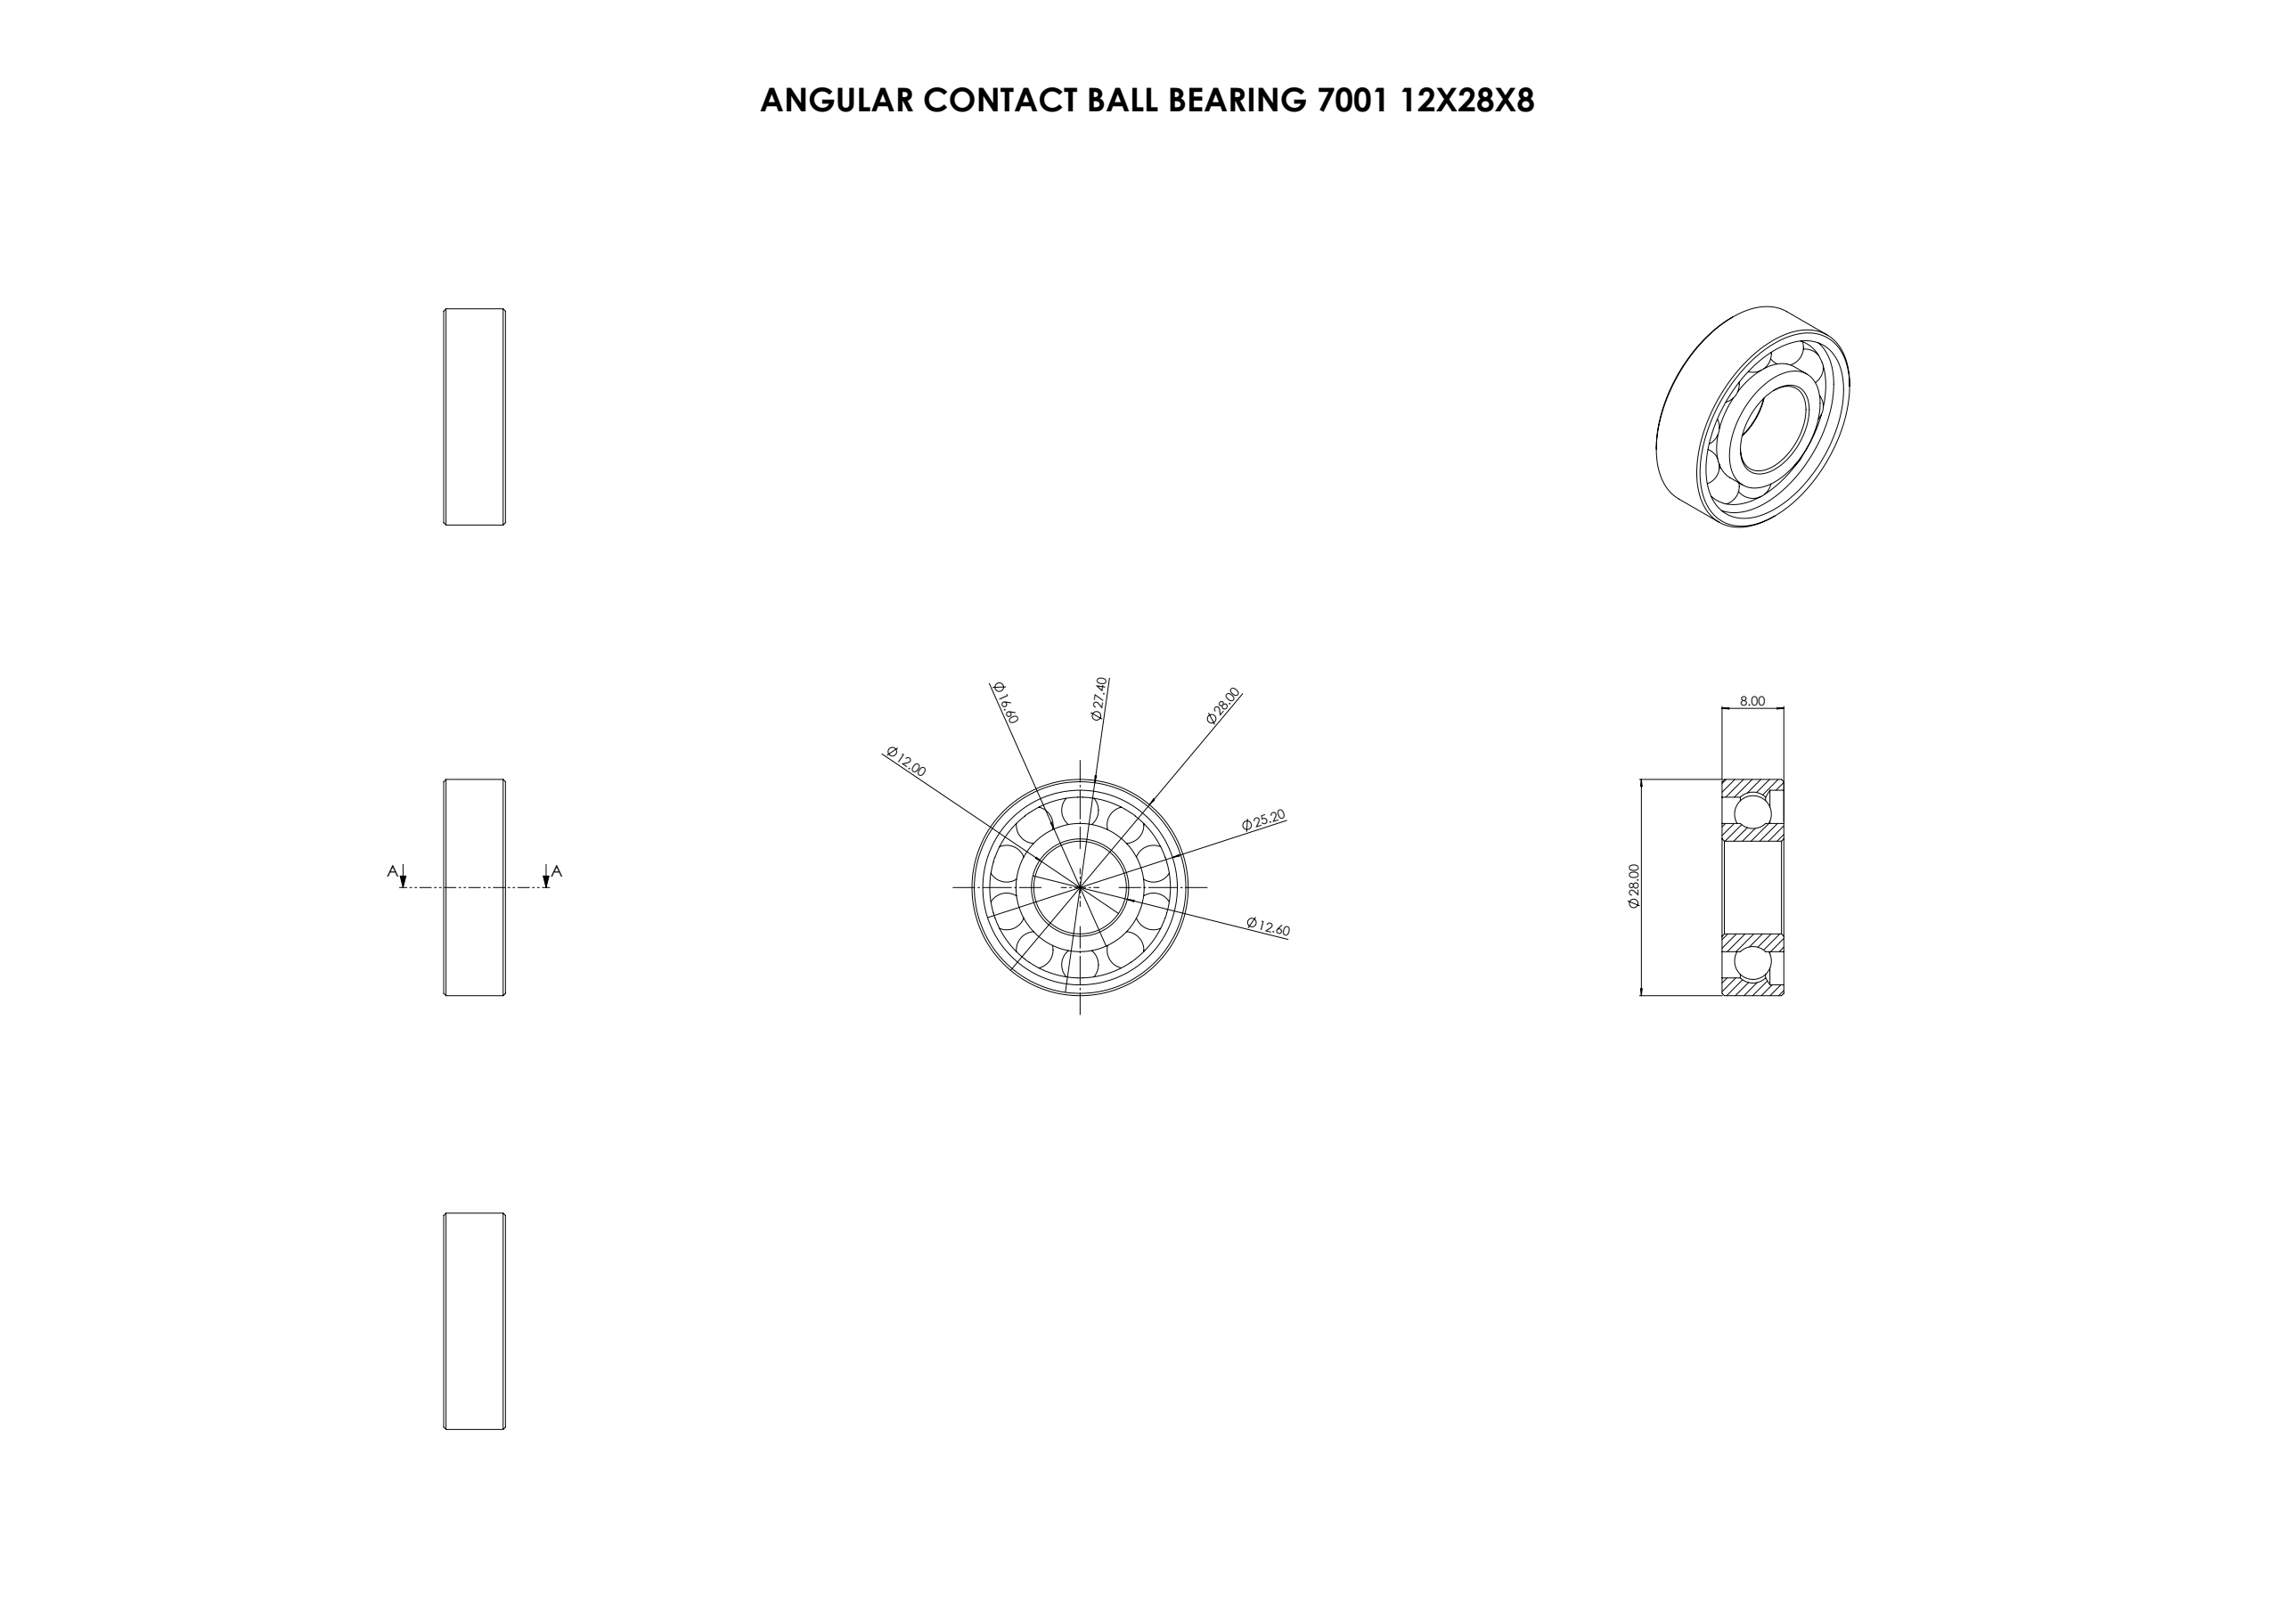
ISO-10303-21;
HEADER;
/* Generated by software containing ST-Developer
 * from STEP Tools, Inc. (www.steptools.com) 
 */

FILE_DESCRIPTION(
/* description */ (''),
/* implementation_level */ '2;1');

FILE_NAME(
/* name */ '06_Angular_Contact_Ball_Bearing_7001_12x28x8.step',
/* time_stamp */ '2026-10-11T09:12:28-07:00',
/* author */ (''),
/* organization */ (''),
/* preprocessor_version */ 'ST-DEVELOPER v20.2',
/* originating_system */ 'Autodesk Translation Framework v15.15.0.0',
/* authorisation */ '');

FILE_SCHEMA (('AUTOMOTIVE_DESIGN { 1 0 10303 214 3 1 1 }'));
ENDSEC;

DATA;
#10=MECHANICAL_DESIGN_GEOMETRIC_PRESENTATION_REPRESENTATION('',(#652),#23254);
#83=SPHERICAL_SURFACE('',#7605,2.38125);
#84=SPHERICAL_SURFACE('',#7635,2.38125);
#85=SPHERICAL_SURFACE('',#7641,2.38125);
#86=SPHERICAL_SURFACE('',#7647,2.38125);
#87=SPHERICAL_SURFACE('',#7653,2.38125);
#88=SPHERICAL_SURFACE('',#7659,2.38125);
#89=SPHERICAL_SURFACE('',#7665,2.38125);
#90=SPHERICAL_SURFACE('',#7671,2.38125);
#91=SPHERICAL_SURFACE('',#7677,2.38125);
#92=SPHERICAL_SURFACE('',#7689,2.38125);
#517=B_SPLINE_CURVE_WITH_KNOTS('',3,(#21115,#21116,#21117,#21118,#21119,
#21120),.UNSPECIFIED.,.F.,.F.,(4,2,4),(0.226218361876484,0.25919316472602,
0.292167967575556),.UNSPECIFIED.);
#518=B_SPLINE_CURVE_WITH_KNOTS('',3,(#21122,#21123,#21124,#21125,#21126,
#21127,#21128,#21129,#21130,#21131,#21132),.UNSPECIFIED.,.F.,.F.,(4,2,3,
2,4),(-0.170336741191592,-0.0873737681171707,0.,0.0873737681171706,0.170336741191592),
 .UNSPECIFIED.);
#519=B_SPLINE_CURVE_WITH_KNOTS('',3,(#21134,#21135,#21136,#21137,#21138,
#21139),.UNSPECIFIED.,.F.,.F.,(4,2,4),(0.958318332016868,0.991720601129839,
1.02512287024281),.UNSPECIFIED.);
#520=B_SPLINE_CURVE_WITH_KNOTS('',3,(#21140,#21141,#21142,#21143,#21144,
#21145,#21146,#21147,#21148,#21149,#21150),.UNSPECIFIED.,.F.,.F.,(4,2,3,
2,4),(-0.170336741191593,-0.0873737681171707,0.,0.0873737681171707,0.170336741191592),
 .UNSPECIFIED.);
#521=B_SPLINE_CURVE_WITH_KNOTS('',3,(#21153,#21154,#21155,#21156,#21157,
#21158),.UNSPECIFIED.,.F.,.F.,(4,2,4),(0.699168310489759,0.727019400778947,
0.754870491068134),.UNSPECIFIED.);
#522=B_SPLINE_CURVE_WITH_KNOTS('',3,(#21160,#21161,#21162,#21163,#21164,
#21165,#21166,#21167,#21168,#21169),.UNSPECIFIED.,.F.,.F.,(4,2,2,2,4),(0.528720639901106,
0.611686436801216,0.699059005116263,0.78643157343131,0.869397370331421),
 .UNSPECIFIED.);
#523=B_SPLINE_CURVE_WITH_KNOTS('',3,(#21171,#21172,#21173,#21174,#21175,
#21176),.UNSPECIFIED.,.F.,.F.,(4,2,4),(0.21448870997046,0.242339800259649,
0.270190890548838),.UNSPECIFIED.);
#524=B_SPLINE_CURVE_WITH_KNOTS('',3,(#21177,#21178,#21179,#21180,#21181,
#21182,#21183,#21184,#21185,#21186),.UNSPECIFIED.,.F.,.F.,(4,2,2,2,4),(0.528720639901106,
0.611686436801217,0.699059005116263,0.78643157343131,0.869397370331421),
 .UNSPECIFIED.);
#525=B_SPLINE_CURVE_WITH_KNOTS('',3,(#21193,#21194,#21195,#21196),
 .UNSPECIFIED.,.F.,.F.,(4,4),(0.991720601129836,1.02512287024281),
 .UNSPECIFIED.);
#526=B_SPLINE_CURVE_WITH_KNOTS('',3,(#21200,#21201,#21202,#21203,#21204,
#21205),.UNSPECIFIED.,.F.,.F.,(4,2,4),(0.958318332016865,0.991720601129836,
1.02512287024281),.UNSPECIFIED.);
#527=B_SPLINE_CURVE_WITH_KNOTS('',3,(#21209,#21210,#21211,#21212,#21213,
#21214),.UNSPECIFIED.,.F.,.F.,(4,2,4),(0.958318332016865,0.991720601129836,
1.02512287024281),.UNSPECIFIED.);
#528=B_SPLINE_CURVE_WITH_KNOTS('',3,(#21218,#21219,#21220,#21221,#21222,
#21223),.UNSPECIFIED.,.F.,.F.,(4,2,4),(0.958318332016865,0.991720601129836,
1.02512287024281),.UNSPECIFIED.);
#529=B_SPLINE_CURVE_WITH_KNOTS('',3,(#21227,#21228,#21229,#21230,#21231,
#21232),.UNSPECIFIED.,.F.,.F.,(4,2,4),(0.958318332016865,0.991720601129836,
1.02512287024281),.UNSPECIFIED.);
#530=B_SPLINE_CURVE_WITH_KNOTS('',3,(#21236,#21237,#21238,#21239,#21240,
#21241),.UNSPECIFIED.,.F.,.F.,(4,2,4),(0.958318332016865,0.991720601129836,
1.02512287024281),.UNSPECIFIED.);
#531=B_SPLINE_CURVE_WITH_KNOTS('',3,(#21246,#21247,#21248,#21249,#21250,
#21251),.UNSPECIFIED.,.F.,.F.,(4,2,4),(0.958318332016865,0.991720601129837,
1.02512287024281),.UNSPECIFIED.);
#532=B_SPLINE_CURVE_WITH_KNOTS('',3,(#21255,#21256,#21257,#21258,#21259,
#21260),.UNSPECIFIED.,.F.,.F.,(4,2,4),(0.958318332016865,0.991720601129836,
1.02512287024281),.UNSPECIFIED.);
#533=B_SPLINE_CURVE_WITH_KNOTS('',3,(#21264,#21265,#21266,#21267,#21268,
#21269),.UNSPECIFIED.,.F.,.F.,(4,2,4),(0.958318332016866,0.99172060112984,
1.02512287024281),.UNSPECIFIED.);
#534=B_SPLINE_CURVE_WITH_KNOTS('',3,(#21272,#21273,#21274,#21275),
 .UNSPECIFIED.,.F.,.F.,(4,4),(0.958318332016865,0.991720601129836),
 .UNSPECIFIED.);
#535=B_SPLINE_CURVE_WITH_KNOTS('',3,(#21279,#21280,#21281,#21282,#21283,
#21284,#21285,#21286,#21287,#21288,#21289),.UNSPECIFIED.,.F.,.F.,(4,2,3,
2,4),(-0.170336741191593,-0.0873737681171707,0.,0.0873737681171707,0.170336741191592),
 .UNSPECIFIED.);
#536=B_SPLINE_CURVE_WITH_KNOTS('',3,(#21294,#21295,#21296,#21297,#21298,
#21299),.UNSPECIFIED.,.F.,.F.,(4,2,4),(0.21448870997046,0.242339800259649,
0.270190890548838),.UNSPECIFIED.);
#537=B_SPLINE_CURVE_WITH_KNOTS('',3,(#21303,#21304,#21305,#21306,#21307,
#21308),.UNSPECIFIED.,.F.,.F.,(4,2,4),(0.21448870997046,0.242339800259649,
0.270190890548838),.UNSPECIFIED.);
#538=B_SPLINE_CURVE_WITH_KNOTS('',3,(#21312,#21313,#21314,#21315,#21316,
#21317),.UNSPECIFIED.,.F.,.F.,(4,2,4),(0.21448870997046,0.242339800259649,
0.270190890548838),.UNSPECIFIED.);
#539=B_SPLINE_CURVE_WITH_KNOTS('',3,(#21321,#21322,#21323,#21324),
 .UNSPECIFIED.,.F.,.F.,(4,4),(0.21448870997046,0.242339800259649),
 .UNSPECIFIED.);
#540=B_SPLINE_CURVE_WITH_KNOTS('',3,(#21329,#21330,#21331,#21332),
 .UNSPECIFIED.,.F.,.F.,(4,4),(0.242339800259649,0.270190890548838),
 .UNSPECIFIED.);
#541=B_SPLINE_CURVE_WITH_KNOTS('',3,(#21336,#21337,#21338,#21339,#21340,
#21341),.UNSPECIFIED.,.F.,.F.,(4,2,4),(0.21448870997046,0.242339800259649,
0.270190890548838),.UNSPECIFIED.);
#542=B_SPLINE_CURVE_WITH_KNOTS('',3,(#21345,#21346,#21347,#21348,#21349,
#21350),.UNSPECIFIED.,.F.,.F.,(4,2,4),(0.21448870997046,0.242339800259649,
0.270190890548838),.UNSPECIFIED.);
#543=B_SPLINE_CURVE_WITH_KNOTS('',3,(#21354,#21355,#21356,#21357,#21358,
#21359),.UNSPECIFIED.,.F.,.F.,(4,2,4),(0.21448870997046,0.242339800259649,
0.270190890548838),.UNSPECIFIED.);
#544=B_SPLINE_CURVE_WITH_KNOTS('',3,(#21363,#21364,#21365,#21366,#21367,
#21368),.UNSPECIFIED.,.F.,.F.,(4,2,4),(0.21448870997046,0.242339800259649,
0.270190890548838),.UNSPECIFIED.);
#545=B_SPLINE_CURVE_WITH_KNOTS('',3,(#21372,#21373,#21374,#21375,#21376,
#21377),.UNSPECIFIED.,.F.,.F.,(4,2,4),(0.21448870997046,0.242339800259649,
0.270190890548838),.UNSPECIFIED.);
#546=B_SPLINE_CURVE_WITH_KNOTS('',3,(#21382,#21383,#21384,#21385,#21386,
#21387,#21388,#21389,#21390,#21391),.UNSPECIFIED.,.F.,.F.,(4,2,2,2,4),(0.528720639901106,
0.611686436801216,0.699059005116263,0.786431573431309,0.869397370331421),
 .UNSPECIFIED.);
#547=B_SPLINE_CURVE_WITH_KNOTS('',3,(#21397,#21398,#21399,#21400,#21401,
#21402),.UNSPECIFIED.,.F.,.F.,(4,2,4),(0.226218361876484,0.259193164726019,
0.292167967575555),.UNSPECIFIED.);
#548=B_SPLINE_CURVE_WITH_KNOTS('',3,(#21403,#21404,#21405,#21406,#21407,
#21408,#21409,#21410,#21411,#21412,#21413),.UNSPECIFIED.,.F.,.F.,(4,2,3,
2,4),(-0.170336741191593,-0.0873737681171707,0.,0.0873737681171706,0.170336741191593),
 .UNSPECIFIED.);
#549=B_SPLINE_CURVE_WITH_KNOTS('',3,(#21415,#21416,#21417,#21418,#21419,
#21420),.UNSPECIFIED.,.F.,.F.,(4,2,4),(0.69916831048976,0.727019400778947,
0.754870491068134),.UNSPECIFIED.);
#550=B_SPLINE_CURVE_WITH_KNOTS('',3,(#21421,#21422,#21423,#21424,#21425,
#21426,#21427,#21428,#21429,#21430),.UNSPECIFIED.,.F.,.F.,(4,2,2,2,4),(0.528720639901105,
0.611686436801216,0.699059005116263,0.786431573431309,0.86939737033142),
 .UNSPECIFIED.);
#551=B_SPLINE_CURVE_WITH_KNOTS('',3,(#21434,#21435,#21436,#21437,#21438,
#21439,#21440,#21441,#21442,#21443,#21444),.UNSPECIFIED.,.F.,.F.,(4,2,3,
2,4),(-0.170336741191592,-0.0873737681171707,0.,0.0873737681171709,0.170336741191593),
 .UNSPECIFIED.);
#552=B_SPLINE_CURVE_WITH_KNOTS('',3,(#21448,#21449,#21450,#21451,#21452,
#21453,#21454,#21455,#21456,#21457),.UNSPECIFIED.,.F.,.F.,(4,2,2,2,4),(0.528720639901106,
0.611686436801216,0.699059005116263,0.78643157343131,0.869397370331421),
 .UNSPECIFIED.);
#553=B_SPLINE_CURVE_WITH_KNOTS('',3,(#21463,#21464,#21465,#21466,#21467,
#21468),.UNSPECIFIED.,.F.,.F.,(4,2,4),(0.226218361876484,0.259193164726019,
0.292167967575555),.UNSPECIFIED.);
#554=B_SPLINE_CURVE_WITH_KNOTS('',3,(#21469,#21470,#21471,#21472,#21473,
#21474,#21475,#21476,#21477,#21478,#21479),.UNSPECIFIED.,.F.,.F.,(4,2,3,
2,4),(-0.170336741191593,-0.0873737681171709,0.,0.0873737681171706,0.170336741191592),
 .UNSPECIFIED.);
#555=B_SPLINE_CURVE_WITH_KNOTS('',3,(#21481,#21482,#21483,#21484,#21485,
#21486),.UNSPECIFIED.,.F.,.F.,(4,2,4),(0.69916831048976,0.727019400778947,
0.754870491068134),.UNSPECIFIED.);
#556=B_SPLINE_CURVE_WITH_KNOTS('',3,(#21487,#21488,#21489,#21490,#21491,
#21492,#21493,#21494,#21495,#21496),.UNSPECIFIED.,.F.,.F.,(4,2,2,2,4),(0.528720639901106,
0.611686436801216,0.699059005116263,0.78643157343131,0.869397370331421),
 .UNSPECIFIED.);
#557=B_SPLINE_CURVE_WITH_KNOTS('',3,(#21500,#21501,#21502,#21503,#21504,
#21505,#21506,#21507,#21508,#21509,#21510),.UNSPECIFIED.,.F.,.F.,(4,2,3,
2,4),(-0.170336741191593,-0.0873737681171707,0.,0.0873737681171706,0.170336741191593),
 .UNSPECIFIED.);
#558=B_SPLINE_CURVE_WITH_KNOTS('',3,(#21514,#21515,#21516,#21517,#21518,
#21519,#21520,#21521,#21522,#21523),.UNSPECIFIED.,.F.,.F.,(4,2,2,2,4),(0.528720639901106,
0.611686436801217,0.699059005116263,0.78643157343131,0.869397370331421),
 .UNSPECIFIED.);
#559=B_SPLINE_CURVE_WITH_KNOTS('',3,(#21529,#21530,#21531,#21532,#21533,
#21534),.UNSPECIFIED.,.F.,.F.,(4,2,4),(0.226218361876484,0.25919316472602,
0.292167967575555),.UNSPECIFIED.);
#560=B_SPLINE_CURVE_WITH_KNOTS('',3,(#21535,#21536,#21537,#21538,#21539,
#21540,#21541,#21542,#21543,#21544,#21545),.UNSPECIFIED.,.F.,.F.,(4,2,3,
2,4),(-0.170336741191592,-0.0873737681171705,0.,0.0873737681171705,0.170336741191593),
 .UNSPECIFIED.);
#561=B_SPLINE_CURVE_WITH_KNOTS('',3,(#21547,#21548,#21549,#21550,#21551,
#21552),.UNSPECIFIED.,.F.,.F.,(4,2,4),(0.699168310489759,0.727019400778946,
0.754870491068134),.UNSPECIFIED.);
#562=B_SPLINE_CURVE_WITH_KNOTS('',3,(#21553,#21554,#21555,#21556,#21557,
#21558,#21559,#21560,#21561,#21562),.UNSPECIFIED.,.F.,.F.,(4,2,2,2,4),(0.528720639901106,
0.611686436801216,0.699059005116263,0.786431573431309,0.86939737033142),
 .UNSPECIFIED.);
#563=B_SPLINE_CURVE_WITH_KNOTS('',3,(#21566,#21567,#21568,#21569,#21570,
#21571,#21572,#21573,#21574,#21575,#21576),.UNSPECIFIED.,.F.,.F.,(4,2,3,
2,4),(-0.170336741191593,-0.0873737681171707,0.,0.0873737681171707,0.170336741191592),
 .UNSPECIFIED.);
#564=B_SPLINE_CURVE_WITH_KNOTS('',3,(#21580,#21581,#21582,#21583,#21584,
#21585,#21586,#21587,#21588,#21589),.UNSPECIFIED.,.F.,.F.,(4,2,2,2,4),(0.528720639901106,
0.611686436801217,0.699059005116263,0.78643157343131,0.869397370331421),
 .UNSPECIFIED.);
#565=B_SPLINE_CURVE_WITH_KNOTS('',3,(#21596,#21597,#21598,#21599),
 .UNSPECIFIED.,.F.,.F.,(4,4),(0.226218361876484,0.259193164726019),
 .UNSPECIFIED.);
#566=B_SPLINE_CURVE_WITH_KNOTS('',3,(#21600,#21601,#21602,#21603,#21604,
#21605,#21606,#21607,#21608,#21609,#21610),.UNSPECIFIED.,.F.,.F.,(4,2,3,
2,4),(-0.170336741191593,-0.0873737681171707,0.,0.0873737681171706,0.170336741191593),
 .UNSPECIFIED.);
#567=B_SPLINE_CURVE_WITH_KNOTS('',3,(#21611,#21612,#21613,#21614),
 .UNSPECIFIED.,.F.,.F.,(4,4),(0.259193164726019,0.292167967575555),
 .UNSPECIFIED.);
#568=B_SPLINE_CURVE_WITH_KNOTS('',3,(#21617,#21618,#21619,#21620),
 .UNSPECIFIED.,.F.,.F.,(4,4),(0.69916831048976,0.727019400778947),
 .UNSPECIFIED.);
#569=B_SPLINE_CURVE_WITH_KNOTS('',3,(#21621,#21622,#21623,#21624,#21625,
#21626,#21627,#21628,#21629,#21630),.UNSPECIFIED.,.F.,.F.,(4,2,2,2,4),(0.528720639901106,
0.611686436801216,0.699059005116263,0.78643157343131,0.869397370331421),
 .UNSPECIFIED.);
#570=B_SPLINE_CURVE_WITH_KNOTS('',3,(#21631,#21632,#21633,#21634),
 .UNSPECIFIED.,.F.,.F.,(4,4),(0.727019400778947,0.754870491068135),
 .UNSPECIFIED.);
#571=B_SPLINE_CURVE_WITH_KNOTS('',3,(#21638,#21639,#21640,#21641,#21642,
#21643,#21644,#21645,#21646,#21647,#21648),.UNSPECIFIED.,.F.,.F.,(4,2,3,
2,4),(-0.170336741191592,-0.0873737681171705,0.,0.0873737681171706,0.170336741191592),
 .UNSPECIFIED.);
#572=B_SPLINE_CURVE_WITH_KNOTS('',3,(#21652,#21653,#21654,#21655,#21656,
#21657,#21658,#21659,#21660,#21661),.UNSPECIFIED.,.F.,.F.,(4,2,2,2,4),(0.528720639901106,
0.611686436801216,0.699059005116263,0.78643157343131,0.869397370331421),
 .UNSPECIFIED.);
#573=B_SPLINE_CURVE_WITH_KNOTS('',3,(#21667,#21668,#21669,#21670,#21671,
#21672),.UNSPECIFIED.,.F.,.F.,(4,2,4),(0.226218361876484,0.25919316472602,
0.292167967575555),.UNSPECIFIED.);
#574=B_SPLINE_CURVE_WITH_KNOTS('',3,(#21673,#21674,#21675,#21676,#21677,
#21678,#21679,#21680,#21681,#21682,#21683),.UNSPECIFIED.,.F.,.F.,(4,2,3,
2,4),(-0.170336741191592,-0.0873737681171707,0.,0.0873737681171706,0.170336741191592),
 .UNSPECIFIED.);
#575=B_SPLINE_CURVE_WITH_KNOTS('',3,(#21685,#21686,#21687,#21688,#21689,
#21690),.UNSPECIFIED.,.F.,.F.,(4,2,4),(0.69916831048976,0.727019400778947,
0.754870491068134),.UNSPECIFIED.);
#576=B_SPLINE_CURVE_WITH_KNOTS('',3,(#21691,#21692,#21693,#21694,#21695,
#21696,#21697,#21698,#21699,#21700),.UNSPECIFIED.,.F.,.F.,(4,2,2,2,4),(0.528720639901106,
0.611686436801216,0.699059005116263,0.78643157343131,0.869397370331421),
 .UNSPECIFIED.);
#577=B_SPLINE_CURVE_WITH_KNOTS('',3,(#21704,#21705,#21706,#21707,#21708,
#21709,#21710,#21711,#21712,#21713,#21714),.UNSPECIFIED.,.F.,.F.,(4,2,3,
2,4),(-0.170336741191592,-0.0873737681171707,0.,0.0873737681171707,0.170336741191593),
 .UNSPECIFIED.);
#578=B_SPLINE_CURVE_WITH_KNOTS('',3,(#21718,#21719,#21720,#21721,#21722,
#21723,#21724,#21725,#21726,#21727),.UNSPECIFIED.,.F.,.F.,(4,2,2,2,4),(0.528720639901106,
0.611686436801217,0.699059005116263,0.786431573431309,0.86939737033142),
 .UNSPECIFIED.);
#579=B_SPLINE_CURVE_WITH_KNOTS('',3,(#21733,#21734,#21735,#21736,#21737,
#21738),.UNSPECIFIED.,.F.,.F.,(4,2,4),(0.226218361876484,0.259193164726019,
0.292167967575555),.UNSPECIFIED.);
#580=B_SPLINE_CURVE_WITH_KNOTS('',3,(#21739,#21740,#21741,#21742,#21743,
#21744,#21745,#21746,#21747,#21748,#21749),.UNSPECIFIED.,.F.,.F.,(4,2,3,
2,4),(-0.170336741191593,-0.0873737681171707,0.,0.0873737681171706,0.170336741191593),
 .UNSPECIFIED.);
#581=B_SPLINE_CURVE_WITH_KNOTS('',3,(#21751,#21752,#21753,#21754,#21755,
#21756),.UNSPECIFIED.,.F.,.F.,(4,2,4),(0.699168310489759,0.727019400778947,
0.754870491068134),.UNSPECIFIED.);
#582=B_SPLINE_CURVE_WITH_KNOTS('',3,(#21757,#21758,#21759,#21760,#21761,
#21762,#21763,#21764,#21765,#21766),.UNSPECIFIED.,.F.,.F.,(4,2,2,2,4),(0.528720639901106,
0.611686436801216,0.699059005116263,0.786431573431309,0.86939737033142),
 .UNSPECIFIED.);
#583=B_SPLINE_CURVE_WITH_KNOTS('',3,(#21770,#21771,#21772,#21773,#21774,
#21775,#21776,#21777,#21778,#21779,#21780),.UNSPECIFIED.,.F.,.F.,(4,2,3,
2,4),(-0.170336741191592,-0.0873737681171702,0.,0.0873737681171704,0.170336741191593),
 .UNSPECIFIED.);
#584=B_SPLINE_CURVE_WITH_KNOTS('',3,(#21784,#21785,#21786,#21787,#21788,
#21789,#21790,#21791,#21792,#21793),.UNSPECIFIED.,.F.,.F.,(4,2,2,2,4),(0.528720639901106,
0.611686436801217,0.699059005116263,0.78643157343131,0.869397370331421),
 .UNSPECIFIED.);
#585=B_SPLINE_CURVE_WITH_KNOTS('',3,(#21799,#21800,#21801,#21802,#21803,
#21804),.UNSPECIFIED.,.F.,.F.,(4,2,4),(0.226218361876484,0.25919316472602,
0.292167967575555),.UNSPECIFIED.);
#586=B_SPLINE_CURVE_WITH_KNOTS('',3,(#21805,#21806,#21807,#21808,#21809,
#21810,#21811,#21812,#21813,#21814,#21815),.UNSPECIFIED.,.F.,.F.,(4,2,3,
2,4),(-0.170336741191593,-0.0873737681171702,0.,0.0873737681171703,0.170336741191593),
 .UNSPECIFIED.);
#587=B_SPLINE_CURVE_WITH_KNOTS('',3,(#21817,#21818,#21819,#21820,#21821,
#21822),.UNSPECIFIED.,.F.,.F.,(4,2,4),(0.699168310489759,0.727019400778947,
0.754870491068134),.UNSPECIFIED.);
#588=B_SPLINE_CURVE_WITH_KNOTS('',3,(#21823,#21824,#21825,#21826,#21827,
#21828,#21829,#21830,#21831,#21832),.UNSPECIFIED.,.F.,.F.,(4,2,2,2,4),(0.528720639901106,
0.611686436801216,0.699059005116263,0.78643157343131,0.869397370331421),
 .UNSPECIFIED.);
#589=B_SPLINE_CURVE_WITH_KNOTS('',3,(#21836,#21837,#21838,#21839,#21840,
#21841,#21842,#21843,#21844,#21845,#21846),.UNSPECIFIED.,.F.,.F.,(4,2,3,
2,4),(-0.170336741191592,-0.0873737681171707,0.,0.0873737681171707,0.170336741191592),
 .UNSPECIFIED.);
#590=B_SPLINE_CURVE_WITH_KNOTS('',3,(#21850,#21851,#21852,#21853,#21854,
#21855,#21856,#21857,#21858,#21859),.UNSPECIFIED.,.F.,.F.,(4,2,2,2,4),(0.528720639901106,
0.611686436801216,0.699059005116263,0.78643157343131,0.869397370331421),
 .UNSPECIFIED.);
#591=B_SPLINE_CURVE_WITH_KNOTS('',3,(#21865,#21866,#21867,#21868,#21869,
#21870),.UNSPECIFIED.,.F.,.F.,(4,2,4),(0.226218361876484,0.259193164726019,
0.292167967575555),.UNSPECIFIED.);
#592=B_SPLINE_CURVE_WITH_KNOTS('',3,(#21871,#21872,#21873,#21874,#21875,
#21876,#21877,#21878,#21879,#21880,#21881),.UNSPECIFIED.,.F.,.F.,(4,2,3,
2,4),(-0.170336741191592,-0.0873737681171707,0.,0.0873737681171706,0.170336741191593),
 .UNSPECIFIED.);
#593=B_SPLINE_CURVE_WITH_KNOTS('',3,(#21883,#21884,#21885,#21886,#21887,
#21888),.UNSPECIFIED.,.F.,.F.,(4,2,4),(0.69916831048976,0.727019400778947,
0.754870491068134),.UNSPECIFIED.);
#594=B_SPLINE_CURVE_WITH_KNOTS('',3,(#21889,#21890,#21891,#21892,#21893,
#21894,#21895,#21896,#21897,#21898),.UNSPECIFIED.,.F.,.F.,(4,2,2,2,4),(0.528720639901105,
0.611686436801216,0.699059005116263,0.786431573431309,0.86939737033142),
 .UNSPECIFIED.);
#595=B_SPLINE_CURVE_WITH_KNOTS('',3,(#21903,#21904,#21905,#21906,#21907,
#21908),.UNSPECIFIED.,.F.,.F.,(4,2,4),(0.226218361876484,0.259193164726019,
0.292167967575555),.UNSPECIFIED.);
#596=B_SPLINE_CURVE_WITH_KNOTS('',3,(#21914,#21915,#21916,#21917,#21918,
#21919,#21920,#21921,#21922,#21923,#21924),.UNSPECIFIED.,.F.,.F.,(4,2,3,
2,4),(-0.170336741191593,-0.0873737681171707,0.,0.0873737681171706,0.170336741191593),
 .UNSPECIFIED.);
#597=B_SPLINE_CURVE_WITH_KNOTS('',3,(#21932,#21933,#21934,#21935,#21936,
#21937),.UNSPECIFIED.,.F.,.F.,(4,2,4),(0.69916831048976,0.727019400778947,
0.754870491068135),.UNSPECIFIED.);
#598=B_SPLINE_CURVE_WITH_KNOTS('',3,(#21940,#21941,#21942,#21943,#21944,
#21945,#21946,#21947,#21948,#21949),.UNSPECIFIED.,.F.,.F.,(4,2,2,2,4),(0.528720639901106,
0.611686436801216,0.699059005116263,0.78643157343131,0.869397370331421),
 .UNSPECIFIED.);
#599=B_SPLINE_CURVE_WITH_KNOTS('',3,(#21954,#21955,#21956,#21957,#21958,
#21959,#21960,#21961,#21962,#21963),.UNSPECIFIED.,.F.,.F.,(4,2,2,2,4),(0.528720639901106,
0.611686436801217,0.699059005116263,0.78643157343131,0.869397370331421),
 .UNSPECIFIED.);
#600=B_SPLINE_CURVE_WITH_KNOTS('',3,(#21964,#21965,#21966,#21967,#21968,
#21969,#21970,#21971,#21972,#21973,#21974),.UNSPECIFIED.,.F.,.F.,(4,2,3,
2,4),(-0.170336741191593,-0.0873737681171707,0.,0.0873737681171707,0.170336741191593),
 .UNSPECIFIED.);
#632=SHAPE_REPRESENTATION_RELATIONSHIP('SRR','None',#23305,#642);
#642=ADVANCED_BREP_SHAPE_REPRESENTATION('',(#662),#23249);
#652=STYLED_ITEM('',(#23462),#662);
#662=MANIFOLD_SOLID_BREP('Body1',#7030);
#743=CONICAL_SURFACE('',#7607,12.15,1.01175638808434);
#744=CONICAL_SURFACE('',#7694,13.85,0.785398163397449);
#745=CONICAL_SURFACE('',#7698,13.85,0.785398163397448);
#746=CONICAL_SURFACE('',#7706,6.15,0.785398163397448);
#747=CONICAL_SURFACE('',#7710,6.15,0.785398163397449);
#760=TOROIDAL_SURFACE('',#7619,10.,2.36);
#761=TOROIDAL_SURFACE('',#7633,10.,2.36);
#762=TOROIDAL_SURFACE('',#7637,10.,2.36);
#763=TOROIDAL_SURFACE('',#7639,10.,2.36);
#764=TOROIDAL_SURFACE('',#7643,10.,2.36);
#765=TOROIDAL_SURFACE('',#7645,10.,2.36);
#766=TOROIDAL_SURFACE('',#7649,10.,2.36);
#767=TOROIDAL_SURFACE('',#7651,10.,2.36);
#768=TOROIDAL_SURFACE('',#7655,10.,2.36);
#769=TOROIDAL_SURFACE('',#7657,10.,2.36);
#770=TOROIDAL_SURFACE('',#7661,10.,2.36);
#771=TOROIDAL_SURFACE('',#7663,10.,2.36);
#772=TOROIDAL_SURFACE('',#7667,10.,2.36);
#773=TOROIDAL_SURFACE('',#7669,10.,2.36);
#774=TOROIDAL_SURFACE('',#7673,10.,2.36);
#775=TOROIDAL_SURFACE('',#7675,10.,2.36);
#776=TOROIDAL_SURFACE('',#7683,10.,2.36);
#777=TOROIDAL_SURFACE('',#7688,10.,2.36);
#778=TOROIDAL_SURFACE('',#7691,10.,2.36);
#779=TOROIDAL_SURFACE('',#7703,10.,2.36);
#814=FACE_BOUND('',#1700,.T.);
#815=FACE_BOUND('',#1701,.T.);
#816=FACE_BOUND('',#1707,.T.);
#817=FACE_BOUND('',#1708,.T.);
#818=FACE_BOUND('',#1712,.T.);
#819=FACE_BOUND('',#1713,.T.);
#820=FACE_BOUND('',#1717,.T.);
#821=FACE_BOUND('',#1718,.T.);
#822=FACE_BOUND('',#1722,.T.);
#823=FACE_BOUND('',#1723,.T.);
#824=FACE_BOUND('',#1727,.T.);
#825=FACE_BOUND('',#1728,.T.);
#826=FACE_BOUND('',#1732,.T.);
#827=FACE_BOUND('',#1733,.T.);
#828=FACE_BOUND('',#1737,.T.);
#829=FACE_BOUND('',#1738,.T.);
#830=FACE_BOUND('',#1742,.T.);
#831=FACE_BOUND('',#1743,.T.);
#832=FACE_BOUND('',#1749,.T.);
#833=FACE_BOUND('',#1750,.T.);
#834=FACE_BOUND('',#1753,.T.);
#835=FACE_BOUND('',#1758,.T.);
#836=FACE_BOUND('',#1762,.T.);
#837=FACE_BOUND('',#1767,.T.);
#948=PLANE('',#7692);
#949=PLANE('',#7700);
#950=PLANE('',#7704);
#951=PLANE('',#7712);
#1270=FACE_OUTER_BOUND('',#1699,.T.);
#1271=FACE_OUTER_BOUND('',#1702,.T.);
#1272=FACE_OUTER_BOUND('',#1703,.T.);
#1273=FACE_OUTER_BOUND('',#1704,.T.);
#1274=FACE_OUTER_BOUND('',#1705,.T.);
#1275=FACE_OUTER_BOUND('',#1706,.T.);
#1276=FACE_OUTER_BOUND('',#1709,.T.);
#1277=FACE_OUTER_BOUND('',#1710,.T.);
#1278=FACE_OUTER_BOUND('',#1711,.T.);
#1279=FACE_OUTER_BOUND('',#1714,.T.);
#1280=FACE_OUTER_BOUND('',#1715,.T.);
#1281=FACE_OUTER_BOUND('',#1716,.T.);
#1282=FACE_OUTER_BOUND('',#1719,.T.);
#1283=FACE_OUTER_BOUND('',#1720,.T.);
#1284=FACE_OUTER_BOUND('',#1721,.T.);
#1285=FACE_OUTER_BOUND('',#1724,.T.);
#1286=FACE_OUTER_BOUND('',#1725,.T.);
#1287=FACE_OUTER_BOUND('',#1726,.T.);
#1288=FACE_OUTER_BOUND('',#1729,.T.);
#1289=FACE_OUTER_BOUND('',#1730,.T.);
#1290=FACE_OUTER_BOUND('',#1731,.T.);
#1291=FACE_OUTER_BOUND('',#1734,.T.);
#1292=FACE_OUTER_BOUND('',#1735,.T.);
#1293=FACE_OUTER_BOUND('',#1736,.T.);
#1294=FACE_OUTER_BOUND('',#1739,.T.);
#1295=FACE_OUTER_BOUND('',#1740,.T.);
#1296=FACE_OUTER_BOUND('',#1741,.T.);
#1297=FACE_OUTER_BOUND('',#1744,.T.);
#1298=FACE_OUTER_BOUND('',#1745,.T.);
#1299=FACE_OUTER_BOUND('',#1746,.T.);
#1300=FACE_OUTER_BOUND('',#1747,.T.);
#1301=FACE_OUTER_BOUND('',#1748,.T.);
#1302=FACE_OUTER_BOUND('',#1751,.T.);
#1303=FACE_OUTER_BOUND('',#1752,.T.);
#1304=FACE_OUTER_BOUND('',#1754,.T.);
#1305=FACE_OUTER_BOUND('',#1755,.T.);
#1306=FACE_OUTER_BOUND('',#1756,.T.);
#1307=FACE_OUTER_BOUND('',#1757,.T.);
#1308=FACE_OUTER_BOUND('',#1759,.T.);
#1309=FACE_OUTER_BOUND('',#1760,.T.);
#1310=FACE_OUTER_BOUND('',#1761,.T.);
#1311=FACE_OUTER_BOUND('',#1763,.T.);
#1312=FACE_OUTER_BOUND('',#1764,.T.);
#1313=FACE_OUTER_BOUND('',#1765,.T.);
#1314=FACE_OUTER_BOUND('',#1766,.T.);
#1699=EDGE_LOOP('',(#5993,#5994));
#1700=EDGE_LOOP('',(#5995,#5996,#5997,#5998));
#1701=EDGE_LOOP('',(#5999,#6000,#6001,#6002));
#1702=EDGE_LOOP('',(#6003,#6004,#6005,#6006,#6007,#6008,#6009,#6010,#6011,
#6012,#6013,#6014,#6015,#6016,#6017,#6018,#6019,#6020,#6021,#6022,#6023,
#6024,#6025,#6026));
#1703=EDGE_LOOP('',(#6027,#6028,#6029,#6030));
#1704=EDGE_LOOP('',(#6031,#6032,#6033,#6034,#6035,#6036,#6037,#6038,#6039,
#6040,#6041,#6042,#6043,#6044,#6045,#6046,#6047,#6048,#6049,#6050,#6051,
#6052,#6053,#6054));
#1705=EDGE_LOOP('',(#6055,#6056,#6057,#6058));
#1706=EDGE_LOOP('',(#6059,#6060));
#1707=EDGE_LOOP('',(#6061,#6062,#6063,#6064));
#1708=EDGE_LOOP('',(#6065,#6066,#6067,#6068));
#1709=EDGE_LOOP('',(#6069,#6070,#6071,#6072));
#1710=EDGE_LOOP('',(#6073,#6074,#6075,#6076));
#1711=EDGE_LOOP('',(#6077,#6078));
#1712=EDGE_LOOP('',(#6079,#6080,#6081,#6082));
#1713=EDGE_LOOP('',(#6083,#6084,#6085,#6086));
#1714=EDGE_LOOP('',(#6087,#6088,#6089,#6090));
#1715=EDGE_LOOP('',(#6091,#6092,#6093,#6094));
#1716=EDGE_LOOP('',(#6095,#6096));
#1717=EDGE_LOOP('',(#6097,#6098,#6099,#6100));
#1718=EDGE_LOOP('',(#6101,#6102,#6103,#6104));
#1719=EDGE_LOOP('',(#6105,#6106,#6107,#6108));
#1720=EDGE_LOOP('',(#6109,#6110,#6111,#6112));
#1721=EDGE_LOOP('',(#6113,#6114));
#1722=EDGE_LOOP('',(#6115,#6116,#6117,#6118,#6119,#6120));
#1723=EDGE_LOOP('',(#6121,#6122,#6123,#6124,#6125,#6126));
#1724=EDGE_LOOP('',(#6127,#6128,#6129,#6130));
#1725=EDGE_LOOP('',(#6131,#6132,#6133,#6134));
#1726=EDGE_LOOP('',(#6135,#6136));
#1727=EDGE_LOOP('',(#6137,#6138,#6139,#6140));
#1728=EDGE_LOOP('',(#6141,#6142,#6143,#6144));
#1729=EDGE_LOOP('',(#6145,#6146,#6147,#6148));
#1730=EDGE_LOOP('',(#6149,#6150,#6151,#6152));
#1731=EDGE_LOOP('',(#6153,#6154));
#1732=EDGE_LOOP('',(#6155,#6156,#6157,#6158));
#1733=EDGE_LOOP('',(#6159,#6160,#6161,#6162));
#1734=EDGE_LOOP('',(#6163,#6164,#6165,#6166));
#1735=EDGE_LOOP('',(#6167,#6168,#6169,#6170));
#1736=EDGE_LOOP('',(#6171,#6172));
#1737=EDGE_LOOP('',(#6173,#6174,#6175,#6176));
#1738=EDGE_LOOP('',(#6177,#6178,#6179,#6180));
#1739=EDGE_LOOP('',(#6181,#6182,#6183,#6184));
#1740=EDGE_LOOP('',(#6185,#6186,#6187,#6188));
#1741=EDGE_LOOP('',(#6189,#6190));
#1742=EDGE_LOOP('',(#6191,#6192,#6193,#6194));
#1743=EDGE_LOOP('',(#6195,#6196,#6197,#6198));
#1744=EDGE_LOOP('',(#6199,#6200,#6201,#6202,#6203,#6204,#6205,#6206,#6207,
#6208,#6209,#6210,#6211,#6212,#6213,#6214,#6215,#6216,#6217,#6218,#6219,
#6220,#6221,#6222));
#1745=EDGE_LOOP('',(#6223,#6224,#6225,#6226));
#1746=EDGE_LOOP('',(#6227,#6228,#6229,#6230,#6231,#6232,#6233,#6234,#6235,
#6236,#6237,#6238,#6239,#6240,#6241,#6242,#6243,#6244,#6245,#6246,#6247,
#6248,#6249,#6250));
#1747=EDGE_LOOP('',(#6251,#6252,#6253,#6254));
#1748=EDGE_LOOP('',(#6255,#6256));
#1749=EDGE_LOOP('',(#6257,#6258,#6259,#6260));
#1750=EDGE_LOOP('',(#6261,#6262,#6263,#6264));
#1751=EDGE_LOOP('',(#6265,#6266,#6267,#6268));
#1752=EDGE_LOOP('',(#6269));
#1753=EDGE_LOOP('',(#6270));
#1754=EDGE_LOOP('',(#6271,#6272,#6273,#6274));
#1755=EDGE_LOOP('',(#6275,#6276,#6277,#6278));
#1756=EDGE_LOOP('',(#6279,#6280,#6281,#6282));
#1757=EDGE_LOOP('',(#6283));
#1758=EDGE_LOOP('',(#6284));
#1759=EDGE_LOOP('',(#6285,#6286,#6287,#6288));
#1760=EDGE_LOOP('',(#6289,#6290,#6291,#6292));
#1761=EDGE_LOOP('',(#6293));
#1762=EDGE_LOOP('',(#6294));
#1763=EDGE_LOOP('',(#6295,#6296,#6297,#6298));
#1764=EDGE_LOOP('',(#6299,#6300,#6301,#6302));
#1765=EDGE_LOOP('',(#6303,#6304,#6305,#6306));
#1766=EDGE_LOOP('',(#6307));
#1767=EDGE_LOOP('',(#6308));
#2025=LINE('',#21191,#2284);
#2026=LINE('',#21326,#2285);
#2027=LINE('',#21911,#2286);
#2028=LINE('',#21928,#2287);
#2029=LINE('',#21982,#2288);
#2030=LINE('',#21986,#2289);
#2031=LINE('',#21990,#2290);
#2032=LINE('',#21995,#2291);
#2033=LINE('',#22002,#2292);
#2034=LINE('',#22006,#2293);
#2035=LINE('',#22010,#2294);
#2284=VECTOR('',#8941,12.15);
#2285=VECTOR('',#8976,8.3);
#2286=VECTOR('',#9089,11.7);
#2287=VECTOR('',#9098,8.3);
#2288=VECTOR('',#9119,13.85);
#2289=VECTOR('',#9124,14.);
#2290=VECTOR('',#9129,13.85);
#2291=VECTOR('',#9136,12.6);
#2292=VECTOR('',#9145,6.15);
#2293=VECTOR('',#9150,6.);
#2294=VECTOR('',#9155,6.15);
#2600=CIRCLE('',#7606,2.38125);
#2601=CIRCLE('',#7608,12.6);
#2602=CIRCLE('',#7609,11.7);
#2603=CIRCLE('',#7610,11.7);
#2604=CIRCLE('',#7611,11.7);
#2605=CIRCLE('',#7612,11.7);
#2606=CIRCLE('',#7613,11.7);
#2607=CIRCLE('',#7614,11.7);
#2608=CIRCLE('',#7615,11.7);
#2609=CIRCLE('',#7616,11.7);
#2610=CIRCLE('',#7617,11.7);
#2611=CIRCLE('',#7618,11.7);
#2612=CIRCLE('',#7620,11.7);
#2613=CIRCLE('',#7622,8.3);
#2614=CIRCLE('',#7623,8.3);
#2615=CIRCLE('',#7624,8.3);
#2616=CIRCLE('',#7625,8.3);
#2617=CIRCLE('',#7626,8.3);
#2618=CIRCLE('',#7627,8.3);
#2619=CIRCLE('',#7628,8.3);
#2620=CIRCLE('',#7629,8.3);
#2621=CIRCLE('',#7630,8.3);
#2622=CIRCLE('',#7631,8.3);
#2623=CIRCLE('',#7632,8.3);
#2624=CIRCLE('',#7634,8.3);
#2625=CIRCLE('',#7636,2.38125);
#2626=CIRCLE('',#7638,11.7);
#2627=CIRCLE('',#7640,8.3);
#2628=CIRCLE('',#7642,2.38125);
#2629=CIRCLE('',#7644,11.7);
#2630=CIRCLE('',#7646,8.3);
#2631=CIRCLE('',#7648,2.38125);
#2632=CIRCLE('',#7650,11.7);
#2633=CIRCLE('',#7652,8.3);
#2634=CIRCLE('',#7654,2.38125);
#2635=CIRCLE('',#7656,11.7);
#2636=CIRCLE('',#7658,8.3);
#2637=CIRCLE('',#7660,2.38125);
#2638=CIRCLE('',#7662,11.7);
#2639=CIRCLE('',#7664,8.3);
#2640=CIRCLE('',#7666,2.38125);
#2641=CIRCLE('',#7668,11.7);
#2642=CIRCLE('',#7670,8.3);
#2643=CIRCLE('',#7672,2.38125);
#2644=CIRCLE('',#7674,11.7);
#2645=CIRCLE('',#7676,8.3);
#2646=CIRCLE('',#7678,2.38125);
#2647=CIRCLE('',#7680,11.7);
#2648=CIRCLE('',#7681,11.7);
#2649=CIRCLE('',#7682,11.7);
#2650=CIRCLE('',#7685,8.3);
#2651=CIRCLE('',#7686,8.3);
#2652=CIRCLE('',#7687,8.3);
#2653=CIRCLE('',#7690,2.38125);
#2654=CIRCLE('',#7693,13.7);
#2655=CIRCLE('',#7695,14.);
#2656=CIRCLE('',#7697,14.);
#2657=CIRCLE('',#7699,13.7);
#2658=CIRCLE('',#7701,12.6);
#2659=CIRCLE('',#7705,6.3);
#2660=CIRCLE('',#7707,6.);
#2661=CIRCLE('',#7709,6.);
#2662=CIRCLE('',#7711,6.3);
#3204=VERTEX_POINT('',#21110);
#3205=VERTEX_POINT('',#21111);
#3206=VERTEX_POINT('',#21113);
#3207=VERTEX_POINT('',#21114);
#3208=VERTEX_POINT('',#21121);
#3209=VERTEX_POINT('',#21133);
#3210=VERTEX_POINT('',#21151);
#3211=VERTEX_POINT('',#21152);
#3212=VERTEX_POINT('',#21159);
#3213=VERTEX_POINT('',#21170);
#3214=VERTEX_POINT('',#21188);
#3215=VERTEX_POINT('',#21190);
#3216=VERTEX_POINT('',#21192);
#3217=VERTEX_POINT('',#21197);
#3218=VERTEX_POINT('',#21199);
#3219=VERTEX_POINT('',#21206);
#3220=VERTEX_POINT('',#21208);
#3221=VERTEX_POINT('',#21215);
#3222=VERTEX_POINT('',#21217);
#3223=VERTEX_POINT('',#21224);
#3224=VERTEX_POINT('',#21226);
#3225=VERTEX_POINT('',#21233);
#3226=VERTEX_POINT('',#21235);
#3227=VERTEX_POINT('',#21243);
#3228=VERTEX_POINT('',#21245);
#3229=VERTEX_POINT('',#21252);
#3230=VERTEX_POINT('',#21254);
#3231=VERTEX_POINT('',#21261);
#3232=VERTEX_POINT('',#21263);
#3233=VERTEX_POINT('',#21270);
#3234=VERTEX_POINT('',#21277);
#3235=VERTEX_POINT('',#21291);
#3236=VERTEX_POINT('',#21293);
#3237=VERTEX_POINT('',#21300);
#3238=VERTEX_POINT('',#21302);
#3239=VERTEX_POINT('',#21309);
#3240=VERTEX_POINT('',#21311);
#3241=VERTEX_POINT('',#21318);
#3242=VERTEX_POINT('',#21320);
#3243=VERTEX_POINT('',#21325);
#3244=VERTEX_POINT('',#21328);
#3245=VERTEX_POINT('',#21333);
#3246=VERTEX_POINT('',#21335);
#3247=VERTEX_POINT('',#21342);
#3248=VERTEX_POINT('',#21344);
#3249=VERTEX_POINT('',#21351);
#3250=VERTEX_POINT('',#21353);
#3251=VERTEX_POINT('',#21360);
#3252=VERTEX_POINT('',#21362);
#3253=VERTEX_POINT('',#21369);
#3254=VERTEX_POINT('',#21371);
#3255=VERTEX_POINT('',#21380);
#3256=VERTEX_POINT('',#21393);
#3257=VERTEX_POINT('',#21394);
#3258=VERTEX_POINT('',#21396);
#3259=VERTEX_POINT('',#21414);
#3260=VERTEX_POINT('',#21432);
#3261=VERTEX_POINT('',#21446);
#3262=VERTEX_POINT('',#21459);
#3263=VERTEX_POINT('',#21460);
#3264=VERTEX_POINT('',#21462);
#3265=VERTEX_POINT('',#21480);
#3266=VERTEX_POINT('',#21498);
#3267=VERTEX_POINT('',#21512);
#3268=VERTEX_POINT('',#21525);
#3269=VERTEX_POINT('',#21526);
#3270=VERTEX_POINT('',#21528);
#3271=VERTEX_POINT('',#21546);
#3272=VERTEX_POINT('',#21564);
#3273=VERTEX_POINT('',#21578);
#3274=VERTEX_POINT('',#21591);
#3275=VERTEX_POINT('',#21592);
#3276=VERTEX_POINT('',#21594);
#3277=VERTEX_POINT('',#21595);
#3278=VERTEX_POINT('',#21615);
#3279=VERTEX_POINT('',#21616);
#3280=VERTEX_POINT('',#21636);
#3281=VERTEX_POINT('',#21650);
#3282=VERTEX_POINT('',#21663);
#3283=VERTEX_POINT('',#21664);
#3284=VERTEX_POINT('',#21666);
#3285=VERTEX_POINT('',#21684);
#3286=VERTEX_POINT('',#21702);
#3287=VERTEX_POINT('',#21716);
#3288=VERTEX_POINT('',#21729);
#3289=VERTEX_POINT('',#21730);
#3290=VERTEX_POINT('',#21732);
#3291=VERTEX_POINT('',#21750);
#3292=VERTEX_POINT('',#21768);
#3293=VERTEX_POINT('',#21782);
#3294=VERTEX_POINT('',#21795);
#3295=VERTEX_POINT('',#21796);
#3296=VERTEX_POINT('',#21798);
#3297=VERTEX_POINT('',#21816);
#3298=VERTEX_POINT('',#21834);
#3299=VERTEX_POINT('',#21848);
#3300=VERTEX_POINT('',#21861);
#3301=VERTEX_POINT('',#21862);
#3302=VERTEX_POINT('',#21864);
#3303=VERTEX_POINT('',#21882);
#3304=VERTEX_POINT('',#21900);
#3305=VERTEX_POINT('',#21902);
#3306=VERTEX_POINT('',#21910);
#3307=VERTEX_POINT('',#21926);
#3308=VERTEX_POINT('',#21929);
#3309=VERTEX_POINT('',#21931);
#3310=VERTEX_POINT('',#21951);
#3311=VERTEX_POINT('',#21952);
#3312=VERTEX_POINT('',#21977);
#3313=VERTEX_POINT('',#21980);
#3314=VERTEX_POINT('',#21984);
#3315=VERTEX_POINT('',#21988);
#3316=VERTEX_POINT('',#21992);
#3317=VERTEX_POINT('',#21998);
#3318=VERTEX_POINT('',#22001);
#3319=VERTEX_POINT('',#22005);
#3320=VERTEX_POINT('',#22009);
#4172=EDGE_CURVE('',#3204,#3205,#2600,.T.);
#4173=EDGE_CURVE('',#3206,#3207,#517,.T.);
#4174=EDGE_CURVE('',#3208,#3206,#518,.T.);
#4175=EDGE_CURVE('',#3209,#3208,#519,.T.);
#4176=EDGE_CURVE('',#3207,#3209,#520,.T.);
#4177=EDGE_CURVE('',#3210,#3211,#521,.T.);
#4178=EDGE_CURVE('',#3212,#3210,#522,.T.);
#4179=EDGE_CURVE('',#3213,#3212,#523,.T.);
#4180=EDGE_CURVE('',#3211,#3213,#524,.T.);
#4181=EDGE_CURVE('',#3214,#3214,#2601,.T.);
#4182=EDGE_CURVE('',#3214,#3215,#2025,.T.);
#4183=EDGE_CURVE('',#3215,#3216,#525,.T.);
#4184=EDGE_CURVE('',#3217,#3216,#2602,.T.);
#4185=EDGE_CURVE('',#3217,#3218,#526,.T.);
#4186=EDGE_CURVE('',#3219,#3218,#2603,.T.);
#4187=EDGE_CURVE('',#3219,#3220,#527,.T.);
#4188=EDGE_CURVE('',#3221,#3220,#2604,.T.);
#4189=EDGE_CURVE('',#3221,#3222,#528,.T.);
#4190=EDGE_CURVE('',#3223,#3222,#2605,.T.);
#4191=EDGE_CURVE('',#3223,#3224,#529,.T.);
#4192=EDGE_CURVE('',#3225,#3224,#2606,.T.);
#4193=EDGE_CURVE('',#3225,#3226,#530,.T.);
#4194=EDGE_CURVE('',#3209,#3226,#2607,.T.);
#4195=EDGE_CURVE('',#3227,#3208,#2608,.T.);
#4196=EDGE_CURVE('',#3227,#3228,#531,.T.);
#4197=EDGE_CURVE('',#3229,#3228,#2609,.T.);
#4198=EDGE_CURVE('',#3229,#3230,#532,.T.);
#4199=EDGE_CURVE('',#3231,#3230,#2610,.T.);
#4200=EDGE_CURVE('',#3231,#3232,#533,.T.);
#4201=EDGE_CURVE('',#3233,#3232,#2611,.T.);
#4202=EDGE_CURVE('',#3233,#3215,#534,.T.);
#4203=EDGE_CURVE('',#3234,#3206,#2612,.T.);
#4204=EDGE_CURVE('',#3234,#3227,#535,.T.);
#4205=EDGE_CURVE('',#3235,#3212,#2613,.T.);
#4206=EDGE_CURVE('',#3235,#3236,#536,.T.);
#4207=EDGE_CURVE('',#3237,#3236,#2614,.T.);
#4208=EDGE_CURVE('',#3237,#3238,#537,.T.);
#4209=EDGE_CURVE('',#3239,#3238,#2615,.T.);
#4210=EDGE_CURVE('',#3239,#3240,#538,.T.);
#4211=EDGE_CURVE('',#3241,#3240,#2616,.T.);
#4212=EDGE_CURVE('',#3241,#3242,#539,.T.);
#4213=EDGE_CURVE('',#3242,#3243,#2026,.T.);
#4214=EDGE_CURVE('',#3243,#3243,#2617,.T.);
#4215=EDGE_CURVE('',#3242,#3244,#540,.T.);
#4216=EDGE_CURVE('',#3245,#3244,#2618,.T.);
#4217=EDGE_CURVE('',#3245,#3246,#541,.T.);
#4218=EDGE_CURVE('',#3247,#3246,#2619,.T.);
#4219=EDGE_CURVE('',#3247,#3248,#542,.T.);
#4220=EDGE_CURVE('',#3249,#3248,#2620,.T.);
#4221=EDGE_CURVE('',#3249,#3250,#543,.T.);
#4222=EDGE_CURVE('',#3251,#3250,#2621,.T.);
#4223=EDGE_CURVE('',#3251,#3252,#544,.T.);
#4224=EDGE_CURVE('',#3253,#3252,#2622,.T.);
#4225=EDGE_CURVE('',#3253,#3254,#545,.T.);
#4226=EDGE_CURVE('',#3213,#3254,#2623,.T.);
#4227=EDGE_CURVE('',#3255,#3210,#2624,.T.);
#4228=EDGE_CURVE('',#3255,#3235,#546,.T.);
#4229=EDGE_CURVE('',#3256,#3257,#2625,.T.);
#4230=EDGE_CURVE('',#3258,#3234,#547,.T.);
#4231=EDGE_CURVE('',#3228,#3258,#548,.T.);
#4232=EDGE_CURVE('',#3259,#3255,#549,.T.);
#4233=EDGE_CURVE('',#3236,#3259,#550,.T.);
#4234=EDGE_CURVE('',#3260,#3258,#2626,.T.);
#4235=EDGE_CURVE('',#3260,#3229,#551,.T.);
#4236=EDGE_CURVE('',#3261,#3259,#2627,.T.);
#4237=EDGE_CURVE('',#3261,#3237,#552,.T.);
#4238=EDGE_CURVE('',#3262,#3263,#2628,.T.);
#4239=EDGE_CURVE('',#3264,#3260,#553,.T.);
#4240=EDGE_CURVE('',#3230,#3264,#554,.T.);
#4241=EDGE_CURVE('',#3265,#3261,#555,.T.);
#4242=EDGE_CURVE('',#3238,#3265,#556,.T.);
#4243=EDGE_CURVE('',#3266,#3264,#2629,.T.);
#4244=EDGE_CURVE('',#3266,#3231,#557,.T.);
#4245=EDGE_CURVE('',#3267,#3265,#2630,.T.);
#4246=EDGE_CURVE('',#3267,#3239,#558,.T.);
#4247=EDGE_CURVE('',#3268,#3269,#2631,.T.);
#4248=EDGE_CURVE('',#3270,#3266,#559,.T.);
#4249=EDGE_CURVE('',#3232,#3270,#560,.T.);
#4250=EDGE_CURVE('',#3271,#3267,#561,.T.);
#4251=EDGE_CURVE('',#3240,#3271,#562,.T.);
#4252=EDGE_CURVE('',#3272,#3270,#2632,.T.);
#4253=EDGE_CURVE('',#3272,#3233,#563,.T.);
#4254=EDGE_CURVE('',#3273,#3271,#2633,.T.);
#4255=EDGE_CURVE('',#3273,#3241,#564,.T.);
#4256=EDGE_CURVE('',#3274,#3275,#2634,.T.);
#4257=EDGE_CURVE('',#3276,#3277,#565,.T.);
#4258=EDGE_CURVE('',#3216,#3276,#566,.T.);
#4259=EDGE_CURVE('',#3277,#3272,#567,.T.);
#4260=EDGE_CURVE('',#3278,#3279,#568,.T.);
#4261=EDGE_CURVE('',#3244,#3278,#569,.T.);
#4262=EDGE_CURVE('',#3279,#3273,#570,.T.);
#4263=EDGE_CURVE('',#3280,#3276,#2635,.T.);
#4264=EDGE_CURVE('',#3280,#3217,#571,.T.);
#4265=EDGE_CURVE('',#3281,#3278,#2636,.T.);
#4266=EDGE_CURVE('',#3281,#3245,#572,.T.);
#4267=EDGE_CURVE('',#3282,#3283,#2637,.T.);
#4268=EDGE_CURVE('',#3284,#3280,#573,.T.);
#4269=EDGE_CURVE('',#3218,#3284,#574,.T.);
#4270=EDGE_CURVE('',#3285,#3281,#575,.T.);
#4271=EDGE_CURVE('',#3246,#3285,#576,.T.);
#4272=EDGE_CURVE('',#3286,#3284,#2638,.T.);
#4273=EDGE_CURVE('',#3286,#3219,#577,.T.);
#4274=EDGE_CURVE('',#3287,#3285,#2639,.T.);
#4275=EDGE_CURVE('',#3287,#3247,#578,.T.);
#4276=EDGE_CURVE('',#3288,#3289,#2640,.T.);
#4277=EDGE_CURVE('',#3290,#3286,#579,.T.);
#4278=EDGE_CURVE('',#3220,#3290,#580,.T.);
#4279=EDGE_CURVE('',#3291,#3287,#581,.T.);
#4280=EDGE_CURVE('',#3248,#3291,#582,.T.);
#4281=EDGE_CURVE('',#3292,#3290,#2641,.T.);
#4282=EDGE_CURVE('',#3292,#3221,#583,.T.);
#4283=EDGE_CURVE('',#3293,#3291,#2642,.T.);
#4284=EDGE_CURVE('',#3293,#3249,#584,.T.);
#4285=EDGE_CURVE('',#3294,#3295,#2643,.T.);
#4286=EDGE_CURVE('',#3296,#3292,#585,.T.);
#4287=EDGE_CURVE('',#3222,#3296,#586,.T.);
#4288=EDGE_CURVE('',#3297,#3293,#587,.T.);
#4289=EDGE_CURVE('',#3250,#3297,#588,.T.);
#4290=EDGE_CURVE('',#3298,#3296,#2644,.T.);
#4291=EDGE_CURVE('',#3298,#3223,#589,.T.);
#4292=EDGE_CURVE('',#3299,#3297,#2645,.T.);
#4293=EDGE_CURVE('',#3299,#3251,#590,.T.);
#4294=EDGE_CURVE('',#3300,#3301,#2646,.T.);
#4295=EDGE_CURVE('',#3302,#3298,#591,.T.);
#4296=EDGE_CURVE('',#3224,#3302,#592,.T.);
#4297=EDGE_CURVE('',#3303,#3299,#593,.T.);
#4298=EDGE_CURVE('',#3252,#3303,#594,.T.);
#4299=EDGE_CURVE('',#3207,#3304,#2647,.T.);
#4300=EDGE_CURVE('',#3304,#3305,#595,.T.);
#4301=EDGE_CURVE('',#3305,#3302,#2648,.T.);
#4302=EDGE_CURVE('',#3277,#3306,#2027,.T.);
#4303=EDGE_CURVE('',#3306,#3306,#2649,.T.);
#4304=EDGE_CURVE('',#3226,#3304,#596,.T.);
#4305=EDGE_CURVE('',#3307,#3307,#2650,.T.);
#4306=EDGE_CURVE('',#3307,#3279,#2028,.T.);
#4307=EDGE_CURVE('',#3211,#3308,#2651,.T.);
#4308=EDGE_CURVE('',#3308,#3309,#597,.T.);
#4309=EDGE_CURVE('',#3309,#3303,#2652,.T.);
#4310=EDGE_CURVE('',#3254,#3308,#598,.T.);
#4311=EDGE_CURVE('',#3310,#3311,#2653,.T.);
#4312=EDGE_CURVE('',#3309,#3253,#599,.T.);
#4313=EDGE_CURVE('',#3305,#3225,#600,.T.);
#4314=EDGE_CURVE('',#3312,#3312,#2654,.T.);
#4315=EDGE_CURVE('',#3313,#3313,#2655,.T.);
#4316=EDGE_CURVE('',#3313,#3312,#2029,.T.);
#4317=EDGE_CURVE('',#3314,#3314,#2656,.T.);
#4318=EDGE_CURVE('',#3314,#3313,#2030,.T.);
#4319=EDGE_CURVE('',#3315,#3315,#2657,.T.);
#4320=EDGE_CURVE('',#3315,#3314,#2031,.T.);
#4321=EDGE_CURVE('',#3316,#3316,#2658,.T.);
#4322=EDGE_CURVE('',#3316,#3214,#2032,.T.);
#4323=EDGE_CURVE('',#3317,#3317,#2659,.T.);
#4324=EDGE_CURVE('',#3317,#3318,#2033,.T.);
#4325=EDGE_CURVE('',#3318,#3318,#2660,.T.);
#4326=EDGE_CURVE('',#3318,#3319,#2034,.T.);
#4327=EDGE_CURVE('',#3319,#3319,#2661,.T.);
#4328=EDGE_CURVE('',#3319,#3320,#2035,.T.);
#4329=EDGE_CURVE('',#3320,#3320,#2662,.T.);
#5993=ORIENTED_EDGE('',*,*,#4172,.T.);
#5994=ORIENTED_EDGE('',*,*,#4172,.F.);
#5995=ORIENTED_EDGE('',*,*,#4173,.F.);
#5996=ORIENTED_EDGE('',*,*,#4174,.F.);
#5997=ORIENTED_EDGE('',*,*,#4175,.F.);
#5998=ORIENTED_EDGE('',*,*,#4176,.F.);
#5999=ORIENTED_EDGE('',*,*,#4177,.F.);
#6000=ORIENTED_EDGE('',*,*,#4178,.F.);
#6001=ORIENTED_EDGE('',*,*,#4179,.F.);
#6002=ORIENTED_EDGE('',*,*,#4180,.F.);
#6003=ORIENTED_EDGE('',*,*,#4181,.T.);
#6004=ORIENTED_EDGE('',*,*,#4182,.T.);
#6005=ORIENTED_EDGE('',*,*,#4183,.T.);
#6006=ORIENTED_EDGE('',*,*,#4184,.F.);
#6007=ORIENTED_EDGE('',*,*,#4185,.T.);
#6008=ORIENTED_EDGE('',*,*,#4186,.F.);
#6009=ORIENTED_EDGE('',*,*,#4187,.T.);
#6010=ORIENTED_EDGE('',*,*,#4188,.F.);
#6011=ORIENTED_EDGE('',*,*,#4189,.T.);
#6012=ORIENTED_EDGE('',*,*,#4190,.F.);
#6013=ORIENTED_EDGE('',*,*,#4191,.T.);
#6014=ORIENTED_EDGE('',*,*,#4192,.F.);
#6015=ORIENTED_EDGE('',*,*,#4193,.T.);
#6016=ORIENTED_EDGE('',*,*,#4194,.F.);
#6017=ORIENTED_EDGE('',*,*,#4175,.T.);
#6018=ORIENTED_EDGE('',*,*,#4195,.F.);
#6019=ORIENTED_EDGE('',*,*,#4196,.T.);
#6020=ORIENTED_EDGE('',*,*,#4197,.F.);
#6021=ORIENTED_EDGE('',*,*,#4198,.T.);
#6022=ORIENTED_EDGE('',*,*,#4199,.F.);
#6023=ORIENTED_EDGE('',*,*,#4200,.T.);
#6024=ORIENTED_EDGE('',*,*,#4201,.F.);
#6025=ORIENTED_EDGE('',*,*,#4202,.T.);
#6026=ORIENTED_EDGE('',*,*,#4182,.F.);
#6027=ORIENTED_EDGE('',*,*,#4174,.T.);
#6028=ORIENTED_EDGE('',*,*,#4203,.F.);
#6029=ORIENTED_EDGE('',*,*,#4204,.T.);
#6030=ORIENTED_EDGE('',*,*,#4195,.T.);
#6031=ORIENTED_EDGE('',*,*,#4179,.T.);
#6032=ORIENTED_EDGE('',*,*,#4205,.F.);
#6033=ORIENTED_EDGE('',*,*,#4206,.T.);
#6034=ORIENTED_EDGE('',*,*,#4207,.F.);
#6035=ORIENTED_EDGE('',*,*,#4208,.T.);
#6036=ORIENTED_EDGE('',*,*,#4209,.F.);
#6037=ORIENTED_EDGE('',*,*,#4210,.T.);
#6038=ORIENTED_EDGE('',*,*,#4211,.F.);
#6039=ORIENTED_EDGE('',*,*,#4212,.T.);
#6040=ORIENTED_EDGE('',*,*,#4213,.T.);
#6041=ORIENTED_EDGE('',*,*,#4214,.T.);
#6042=ORIENTED_EDGE('',*,*,#4213,.F.);
#6043=ORIENTED_EDGE('',*,*,#4215,.T.);
#6044=ORIENTED_EDGE('',*,*,#4216,.F.);
#6045=ORIENTED_EDGE('',*,*,#4217,.T.);
#6046=ORIENTED_EDGE('',*,*,#4218,.F.);
#6047=ORIENTED_EDGE('',*,*,#4219,.T.);
#6048=ORIENTED_EDGE('',*,*,#4220,.F.);
#6049=ORIENTED_EDGE('',*,*,#4221,.T.);
#6050=ORIENTED_EDGE('',*,*,#4222,.F.);
#6051=ORIENTED_EDGE('',*,*,#4223,.T.);
#6052=ORIENTED_EDGE('',*,*,#4224,.F.);
#6053=ORIENTED_EDGE('',*,*,#4225,.T.);
#6054=ORIENTED_EDGE('',*,*,#4226,.F.);
#6055=ORIENTED_EDGE('',*,*,#4178,.T.);
#6056=ORIENTED_EDGE('',*,*,#4227,.F.);
#6057=ORIENTED_EDGE('',*,*,#4228,.T.);
#6058=ORIENTED_EDGE('',*,*,#4205,.T.);
#6059=ORIENTED_EDGE('',*,*,#4229,.T.);
#6060=ORIENTED_EDGE('',*,*,#4229,.F.);
#6061=ORIENTED_EDGE('',*,*,#4230,.F.);
#6062=ORIENTED_EDGE('',*,*,#4231,.F.);
#6063=ORIENTED_EDGE('',*,*,#4196,.F.);
#6064=ORIENTED_EDGE('',*,*,#4204,.F.);
#6065=ORIENTED_EDGE('',*,*,#4232,.F.);
#6066=ORIENTED_EDGE('',*,*,#4233,.F.);
#6067=ORIENTED_EDGE('',*,*,#4206,.F.);
#6068=ORIENTED_EDGE('',*,*,#4228,.F.);
#6069=ORIENTED_EDGE('',*,*,#4231,.T.);
#6070=ORIENTED_EDGE('',*,*,#4234,.F.);
#6071=ORIENTED_EDGE('',*,*,#4235,.T.);
#6072=ORIENTED_EDGE('',*,*,#4197,.T.);
#6073=ORIENTED_EDGE('',*,*,#4233,.T.);
#6074=ORIENTED_EDGE('',*,*,#4236,.F.);
#6075=ORIENTED_EDGE('',*,*,#4237,.T.);
#6076=ORIENTED_EDGE('',*,*,#4207,.T.);
#6077=ORIENTED_EDGE('',*,*,#4238,.T.);
#6078=ORIENTED_EDGE('',*,*,#4238,.F.);
#6079=ORIENTED_EDGE('',*,*,#4239,.F.);
#6080=ORIENTED_EDGE('',*,*,#4240,.F.);
#6081=ORIENTED_EDGE('',*,*,#4198,.F.);
#6082=ORIENTED_EDGE('',*,*,#4235,.F.);
#6083=ORIENTED_EDGE('',*,*,#4241,.F.);
#6084=ORIENTED_EDGE('',*,*,#4242,.F.);
#6085=ORIENTED_EDGE('',*,*,#4208,.F.);
#6086=ORIENTED_EDGE('',*,*,#4237,.F.);
#6087=ORIENTED_EDGE('',*,*,#4240,.T.);
#6088=ORIENTED_EDGE('',*,*,#4243,.F.);
#6089=ORIENTED_EDGE('',*,*,#4244,.T.);
#6090=ORIENTED_EDGE('',*,*,#4199,.T.);
#6091=ORIENTED_EDGE('',*,*,#4242,.T.);
#6092=ORIENTED_EDGE('',*,*,#4245,.F.);
#6093=ORIENTED_EDGE('',*,*,#4246,.T.);
#6094=ORIENTED_EDGE('',*,*,#4209,.T.);
#6095=ORIENTED_EDGE('',*,*,#4247,.T.);
#6096=ORIENTED_EDGE('',*,*,#4247,.F.);
#6097=ORIENTED_EDGE('',*,*,#4248,.F.);
#6098=ORIENTED_EDGE('',*,*,#4249,.F.);
#6099=ORIENTED_EDGE('',*,*,#4200,.F.);
#6100=ORIENTED_EDGE('',*,*,#4244,.F.);
#6101=ORIENTED_EDGE('',*,*,#4250,.F.);
#6102=ORIENTED_EDGE('',*,*,#4251,.F.);
#6103=ORIENTED_EDGE('',*,*,#4210,.F.);
#6104=ORIENTED_EDGE('',*,*,#4246,.F.);
#6105=ORIENTED_EDGE('',*,*,#4249,.T.);
#6106=ORIENTED_EDGE('',*,*,#4252,.F.);
#6107=ORIENTED_EDGE('',*,*,#4253,.T.);
#6108=ORIENTED_EDGE('',*,*,#4201,.T.);
#6109=ORIENTED_EDGE('',*,*,#4251,.T.);
#6110=ORIENTED_EDGE('',*,*,#4254,.F.);
#6111=ORIENTED_EDGE('',*,*,#4255,.T.);
#6112=ORIENTED_EDGE('',*,*,#4211,.T.);
#6113=ORIENTED_EDGE('',*,*,#4256,.T.);
#6114=ORIENTED_EDGE('',*,*,#4256,.F.);
#6115=ORIENTED_EDGE('',*,*,#4257,.F.);
#6116=ORIENTED_EDGE('',*,*,#4258,.F.);
#6117=ORIENTED_EDGE('',*,*,#4183,.F.);
#6118=ORIENTED_EDGE('',*,*,#4202,.F.);
#6119=ORIENTED_EDGE('',*,*,#4253,.F.);
#6120=ORIENTED_EDGE('',*,*,#4259,.F.);
#6121=ORIENTED_EDGE('',*,*,#4260,.F.);
#6122=ORIENTED_EDGE('',*,*,#4261,.F.);
#6123=ORIENTED_EDGE('',*,*,#4215,.F.);
#6124=ORIENTED_EDGE('',*,*,#4212,.F.);
#6125=ORIENTED_EDGE('',*,*,#4255,.F.);
#6126=ORIENTED_EDGE('',*,*,#4262,.F.);
#6127=ORIENTED_EDGE('',*,*,#4258,.T.);
#6128=ORIENTED_EDGE('',*,*,#4263,.F.);
#6129=ORIENTED_EDGE('',*,*,#4264,.T.);
#6130=ORIENTED_EDGE('',*,*,#4184,.T.);
#6131=ORIENTED_EDGE('',*,*,#4261,.T.);
#6132=ORIENTED_EDGE('',*,*,#4265,.F.);
#6133=ORIENTED_EDGE('',*,*,#4266,.T.);
#6134=ORIENTED_EDGE('',*,*,#4216,.T.);
#6135=ORIENTED_EDGE('',*,*,#4267,.T.);
#6136=ORIENTED_EDGE('',*,*,#4267,.F.);
#6137=ORIENTED_EDGE('',*,*,#4268,.F.);
#6138=ORIENTED_EDGE('',*,*,#4269,.F.);
#6139=ORIENTED_EDGE('',*,*,#4185,.F.);
#6140=ORIENTED_EDGE('',*,*,#4264,.F.);
#6141=ORIENTED_EDGE('',*,*,#4270,.F.);
#6142=ORIENTED_EDGE('',*,*,#4271,.F.);
#6143=ORIENTED_EDGE('',*,*,#4217,.F.);
#6144=ORIENTED_EDGE('',*,*,#4266,.F.);
#6145=ORIENTED_EDGE('',*,*,#4269,.T.);
#6146=ORIENTED_EDGE('',*,*,#4272,.F.);
#6147=ORIENTED_EDGE('',*,*,#4273,.T.);
#6148=ORIENTED_EDGE('',*,*,#4186,.T.);
#6149=ORIENTED_EDGE('',*,*,#4271,.T.);
#6150=ORIENTED_EDGE('',*,*,#4274,.F.);
#6151=ORIENTED_EDGE('',*,*,#4275,.T.);
#6152=ORIENTED_EDGE('',*,*,#4218,.T.);
#6153=ORIENTED_EDGE('',*,*,#4276,.T.);
#6154=ORIENTED_EDGE('',*,*,#4276,.F.);
#6155=ORIENTED_EDGE('',*,*,#4277,.F.);
#6156=ORIENTED_EDGE('',*,*,#4278,.F.);
#6157=ORIENTED_EDGE('',*,*,#4187,.F.);
#6158=ORIENTED_EDGE('',*,*,#4273,.F.);
#6159=ORIENTED_EDGE('',*,*,#4279,.F.);
#6160=ORIENTED_EDGE('',*,*,#4280,.F.);
#6161=ORIENTED_EDGE('',*,*,#4219,.F.);
#6162=ORIENTED_EDGE('',*,*,#4275,.F.);
#6163=ORIENTED_EDGE('',*,*,#4278,.T.);
#6164=ORIENTED_EDGE('',*,*,#4281,.F.);
#6165=ORIENTED_EDGE('',*,*,#4282,.T.);
#6166=ORIENTED_EDGE('',*,*,#4188,.T.);
#6167=ORIENTED_EDGE('',*,*,#4280,.T.);
#6168=ORIENTED_EDGE('',*,*,#4283,.F.);
#6169=ORIENTED_EDGE('',*,*,#4284,.T.);
#6170=ORIENTED_EDGE('',*,*,#4220,.T.);
#6171=ORIENTED_EDGE('',*,*,#4285,.T.);
#6172=ORIENTED_EDGE('',*,*,#4285,.F.);
#6173=ORIENTED_EDGE('',*,*,#4286,.F.);
#6174=ORIENTED_EDGE('',*,*,#4287,.F.);
#6175=ORIENTED_EDGE('',*,*,#4189,.F.);
#6176=ORIENTED_EDGE('',*,*,#4282,.F.);
#6177=ORIENTED_EDGE('',*,*,#4288,.F.);
#6178=ORIENTED_EDGE('',*,*,#4289,.F.);
#6179=ORIENTED_EDGE('',*,*,#4221,.F.);
#6180=ORIENTED_EDGE('',*,*,#4284,.F.);
#6181=ORIENTED_EDGE('',*,*,#4287,.T.);
#6182=ORIENTED_EDGE('',*,*,#4290,.F.);
#6183=ORIENTED_EDGE('',*,*,#4291,.T.);
#6184=ORIENTED_EDGE('',*,*,#4190,.T.);
#6185=ORIENTED_EDGE('',*,*,#4289,.T.);
#6186=ORIENTED_EDGE('',*,*,#4292,.F.);
#6187=ORIENTED_EDGE('',*,*,#4293,.T.);
#6188=ORIENTED_EDGE('',*,*,#4222,.T.);
#6189=ORIENTED_EDGE('',*,*,#4294,.T.);
#6190=ORIENTED_EDGE('',*,*,#4294,.F.);
#6191=ORIENTED_EDGE('',*,*,#4191,.F.);
#6192=ORIENTED_EDGE('',*,*,#4291,.F.);
#6193=ORIENTED_EDGE('',*,*,#4295,.F.);
#6194=ORIENTED_EDGE('',*,*,#4296,.F.);
#6195=ORIENTED_EDGE('',*,*,#4223,.F.);
#6196=ORIENTED_EDGE('',*,*,#4293,.F.);
#6197=ORIENTED_EDGE('',*,*,#4297,.F.);
#6198=ORIENTED_EDGE('',*,*,#4298,.F.);
#6199=ORIENTED_EDGE('',*,*,#4173,.T.);
#6200=ORIENTED_EDGE('',*,*,#4299,.T.);
#6201=ORIENTED_EDGE('',*,*,#4300,.T.);
#6202=ORIENTED_EDGE('',*,*,#4301,.T.);
#6203=ORIENTED_EDGE('',*,*,#4295,.T.);
#6204=ORIENTED_EDGE('',*,*,#4290,.T.);
#6205=ORIENTED_EDGE('',*,*,#4286,.T.);
#6206=ORIENTED_EDGE('',*,*,#4281,.T.);
#6207=ORIENTED_EDGE('',*,*,#4277,.T.);
#6208=ORIENTED_EDGE('',*,*,#4272,.T.);
#6209=ORIENTED_EDGE('',*,*,#4268,.T.);
#6210=ORIENTED_EDGE('',*,*,#4263,.T.);
#6211=ORIENTED_EDGE('',*,*,#4257,.T.);
#6212=ORIENTED_EDGE('',*,*,#4302,.T.);
#6213=ORIENTED_EDGE('',*,*,#4303,.F.);
#6214=ORIENTED_EDGE('',*,*,#4302,.F.);
#6215=ORIENTED_EDGE('',*,*,#4259,.T.);
#6216=ORIENTED_EDGE('',*,*,#4252,.T.);
#6217=ORIENTED_EDGE('',*,*,#4248,.T.);
#6218=ORIENTED_EDGE('',*,*,#4243,.T.);
#6219=ORIENTED_EDGE('',*,*,#4239,.T.);
#6220=ORIENTED_EDGE('',*,*,#4234,.T.);
#6221=ORIENTED_EDGE('',*,*,#4230,.T.);
#6222=ORIENTED_EDGE('',*,*,#4203,.T.);
#6223=ORIENTED_EDGE('',*,*,#4176,.T.);
#6224=ORIENTED_EDGE('',*,*,#4194,.T.);
#6225=ORIENTED_EDGE('',*,*,#4304,.T.);
#6226=ORIENTED_EDGE('',*,*,#4299,.F.);
#6227=ORIENTED_EDGE('',*,*,#4305,.F.);
#6228=ORIENTED_EDGE('',*,*,#4306,.T.);
#6229=ORIENTED_EDGE('',*,*,#4262,.T.);
#6230=ORIENTED_EDGE('',*,*,#4254,.T.);
#6231=ORIENTED_EDGE('',*,*,#4250,.T.);
#6232=ORIENTED_EDGE('',*,*,#4245,.T.);
#6233=ORIENTED_EDGE('',*,*,#4241,.T.);
#6234=ORIENTED_EDGE('',*,*,#4236,.T.);
#6235=ORIENTED_EDGE('',*,*,#4232,.T.);
#6236=ORIENTED_EDGE('',*,*,#4227,.T.);
#6237=ORIENTED_EDGE('',*,*,#4177,.T.);
#6238=ORIENTED_EDGE('',*,*,#4307,.T.);
#6239=ORIENTED_EDGE('',*,*,#4308,.T.);
#6240=ORIENTED_EDGE('',*,*,#4309,.T.);
#6241=ORIENTED_EDGE('',*,*,#4297,.T.);
#6242=ORIENTED_EDGE('',*,*,#4292,.T.);
#6243=ORIENTED_EDGE('',*,*,#4288,.T.);
#6244=ORIENTED_EDGE('',*,*,#4283,.T.);
#6245=ORIENTED_EDGE('',*,*,#4279,.T.);
#6246=ORIENTED_EDGE('',*,*,#4274,.T.);
#6247=ORIENTED_EDGE('',*,*,#4270,.T.);
#6248=ORIENTED_EDGE('',*,*,#4265,.T.);
#6249=ORIENTED_EDGE('',*,*,#4260,.T.);
#6250=ORIENTED_EDGE('',*,*,#4306,.F.);
#6251=ORIENTED_EDGE('',*,*,#4180,.T.);
#6252=ORIENTED_EDGE('',*,*,#4226,.T.);
#6253=ORIENTED_EDGE('',*,*,#4310,.T.);
#6254=ORIENTED_EDGE('',*,*,#4307,.F.);
#6255=ORIENTED_EDGE('',*,*,#4311,.T.);
#6256=ORIENTED_EDGE('',*,*,#4311,.F.);
#6257=ORIENTED_EDGE('',*,*,#4310,.F.);
#6258=ORIENTED_EDGE('',*,*,#4225,.F.);
#6259=ORIENTED_EDGE('',*,*,#4312,.F.);
#6260=ORIENTED_EDGE('',*,*,#4308,.F.);
#6261=ORIENTED_EDGE('',*,*,#4304,.F.);
#6262=ORIENTED_EDGE('',*,*,#4193,.F.);
#6263=ORIENTED_EDGE('',*,*,#4313,.F.);
#6264=ORIENTED_EDGE('',*,*,#4300,.F.);
#6265=ORIENTED_EDGE('',*,*,#4296,.T.);
#6266=ORIENTED_EDGE('',*,*,#4301,.F.);
#6267=ORIENTED_EDGE('',*,*,#4313,.T.);
#6268=ORIENTED_EDGE('',*,*,#4192,.T.);
#6269=ORIENTED_EDGE('',*,*,#4314,.F.);
#6270=ORIENTED_EDGE('',*,*,#4303,.T.);
#6271=ORIENTED_EDGE('',*,*,#4315,.F.);
#6272=ORIENTED_EDGE('',*,*,#4316,.T.);
#6273=ORIENTED_EDGE('',*,*,#4314,.T.);
#6274=ORIENTED_EDGE('',*,*,#4316,.F.);
#6275=ORIENTED_EDGE('',*,*,#4317,.F.);
#6276=ORIENTED_EDGE('',*,*,#4318,.T.);
#6277=ORIENTED_EDGE('',*,*,#4315,.T.);
#6278=ORIENTED_EDGE('',*,*,#4318,.F.);
#6279=ORIENTED_EDGE('',*,*,#4319,.F.);
#6280=ORIENTED_EDGE('',*,*,#4320,.T.);
#6281=ORIENTED_EDGE('',*,*,#4317,.T.);
#6282=ORIENTED_EDGE('',*,*,#4320,.F.);
#6283=ORIENTED_EDGE('',*,*,#4319,.T.);
#6284=ORIENTED_EDGE('',*,*,#4321,.F.);
#6285=ORIENTED_EDGE('',*,*,#4321,.T.);
#6286=ORIENTED_EDGE('',*,*,#4322,.T.);
#6287=ORIENTED_EDGE('',*,*,#4181,.F.);
#6288=ORIENTED_EDGE('',*,*,#4322,.F.);
#6289=ORIENTED_EDGE('',*,*,#4298,.T.);
#6290=ORIENTED_EDGE('',*,*,#4309,.F.);
#6291=ORIENTED_EDGE('',*,*,#4312,.T.);
#6292=ORIENTED_EDGE('',*,*,#4224,.T.);
#6293=ORIENTED_EDGE('',*,*,#4305,.T.);
#6294=ORIENTED_EDGE('',*,*,#4323,.F.);
#6295=ORIENTED_EDGE('',*,*,#4323,.T.);
#6296=ORIENTED_EDGE('',*,*,#4324,.T.);
#6297=ORIENTED_EDGE('',*,*,#4325,.F.);
#6298=ORIENTED_EDGE('',*,*,#4324,.F.);
#6299=ORIENTED_EDGE('',*,*,#4325,.T.);
#6300=ORIENTED_EDGE('',*,*,#4326,.T.);
#6301=ORIENTED_EDGE('',*,*,#4327,.F.);
#6302=ORIENTED_EDGE('',*,*,#4326,.F.);
#6303=ORIENTED_EDGE('',*,*,#4327,.T.);
#6304=ORIENTED_EDGE('',*,*,#4328,.T.);
#6305=ORIENTED_EDGE('',*,*,#4329,.F.);
#6306=ORIENTED_EDGE('',*,*,#4328,.F.);
#6307=ORIENTED_EDGE('',*,*,#4214,.F.);
#6308=ORIENTED_EDGE('',*,*,#4329,.T.);
#6605=CYLINDRICAL_SURFACE('',#7621,8.3);
#6606=CYLINDRICAL_SURFACE('',#7679,11.7);
#6607=CYLINDRICAL_SURFACE('',#7684,8.3);
#6608=CYLINDRICAL_SURFACE('',#7696,14.);
#6609=CYLINDRICAL_SURFACE('',#7702,12.6);
#6610=CYLINDRICAL_SURFACE('',#7708,6.);
#6921=ADVANCED_FACE('',(#1270,#814,#815),#83,.T.);
#6922=ADVANCED_FACE('',(#1271),#743,.F.);
#6923=ADVANCED_FACE('',(#1272),#760,.F.);
#6924=ADVANCED_FACE('',(#1273),#6605,.T.);
#6925=ADVANCED_FACE('',(#1274),#761,.F.);
#6926=ADVANCED_FACE('',(#1275,#816,#817),#84,.T.);
#6927=ADVANCED_FACE('',(#1276),#762,.F.);
#6928=ADVANCED_FACE('',(#1277),#763,.F.);
#6929=ADVANCED_FACE('',(#1278,#818,#819),#85,.T.);
#6930=ADVANCED_FACE('',(#1279),#764,.F.);
#6931=ADVANCED_FACE('',(#1280),#765,.F.);
#6932=ADVANCED_FACE('',(#1281,#820,#821),#86,.T.);
#6933=ADVANCED_FACE('',(#1282),#766,.F.);
#6934=ADVANCED_FACE('',(#1283),#767,.F.);
#6935=ADVANCED_FACE('',(#1284,#822,#823),#87,.T.);
#6936=ADVANCED_FACE('',(#1285),#768,.F.);
#6937=ADVANCED_FACE('',(#1286),#769,.F.);
#6938=ADVANCED_FACE('',(#1287,#824,#825),#88,.T.);
#6939=ADVANCED_FACE('',(#1288),#770,.F.);
#6940=ADVANCED_FACE('',(#1289),#771,.F.);
#6941=ADVANCED_FACE('',(#1290,#826,#827),#89,.T.);
#6942=ADVANCED_FACE('',(#1291),#772,.F.);
#6943=ADVANCED_FACE('',(#1292),#773,.F.);
#6944=ADVANCED_FACE('',(#1293,#828,#829),#90,.T.);
#6945=ADVANCED_FACE('',(#1294),#774,.F.);
#6946=ADVANCED_FACE('',(#1295),#775,.F.);
#6947=ADVANCED_FACE('',(#1296,#830,#831),#91,.T.);
#6948=ADVANCED_FACE('',(#1297),#6606,.F.);
#6949=ADVANCED_FACE('',(#1298),#776,.F.);
#6950=ADVANCED_FACE('',(#1299),#6607,.T.);
#6951=ADVANCED_FACE('',(#1300),#777,.F.);
#6952=ADVANCED_FACE('',(#1301,#832,#833),#92,.T.);
#6953=ADVANCED_FACE('',(#1302),#778,.F.);
#6954=ADVANCED_FACE('',(#1303,#834),#948,.T.);
#6955=ADVANCED_FACE('',(#1304),#744,.T.);
#6956=ADVANCED_FACE('',(#1305),#6608,.T.);
#6957=ADVANCED_FACE('',(#1306),#745,.T.);
#6958=ADVANCED_FACE('',(#1307,#835),#949,.T.);
#6959=ADVANCED_FACE('',(#1308),#6609,.F.);
#6960=ADVANCED_FACE('',(#1309),#779,.F.);
#6961=ADVANCED_FACE('',(#1310,#836),#950,.T.);
#6962=ADVANCED_FACE('',(#1311),#746,.F.);
#6963=ADVANCED_FACE('',(#1312),#6610,.F.);
#6964=ADVANCED_FACE('',(#1313),#747,.F.);
#6965=ADVANCED_FACE('',(#1314,#837),#951,.T.);
#7030=CLOSED_SHELL('',(#6921,#6922,#6923,#6924,#6925,#6926,#6927,#6928,
#6929,#6930,#6931,#6932,#6933,#6934,#6935,#6936,#6937,#6938,#6939,#6940,
#6941,#6942,#6943,#6944,#6945,#6946,#6947,#6948,#6949,#6950,#6951,#6952,
#6953,#6954,#6955,#6956,#6957,#6958,#6959,#6960,#6961,#6962,#6963,#6964,
#6965));
#7604=AXIS2_PLACEMENT_3D('',#21108,#8931,#8932);
#7605=AXIS2_PLACEMENT_3D('',#21109,#8933,#8934);
#7606=AXIS2_PLACEMENT_3D('',#21112,#8935,#8936);
#7607=AXIS2_PLACEMENT_3D('',#21187,#8937,#8938);
#7608=AXIS2_PLACEMENT_3D('',#21189,#8939,#8940);
#7609=AXIS2_PLACEMENT_3D('',#21198,#8942,#8943);
#7610=AXIS2_PLACEMENT_3D('',#21207,#8944,#8945);
#7611=AXIS2_PLACEMENT_3D('',#21216,#8946,#8947);
#7612=AXIS2_PLACEMENT_3D('',#21225,#8948,#8949);
#7613=AXIS2_PLACEMENT_3D('',#21234,#8950,#8951);
#7614=AXIS2_PLACEMENT_3D('',#21242,#8952,#8953);
#7615=AXIS2_PLACEMENT_3D('',#21244,#8954,#8955);
#7616=AXIS2_PLACEMENT_3D('',#21253,#8956,#8957);
#7617=AXIS2_PLACEMENT_3D('',#21262,#8958,#8959);
#7618=AXIS2_PLACEMENT_3D('',#21271,#8960,#8961);
#7619=AXIS2_PLACEMENT_3D('',#21276,#8962,#8963);
#7620=AXIS2_PLACEMENT_3D('',#21278,#8964,#8965);
#7621=AXIS2_PLACEMENT_3D('',#21290,#8966,#8967);
#7622=AXIS2_PLACEMENT_3D('',#21292,#8968,#8969);
#7623=AXIS2_PLACEMENT_3D('',#21301,#8970,#8971);
#7624=AXIS2_PLACEMENT_3D('',#21310,#8972,#8973);
#7625=AXIS2_PLACEMENT_3D('',#21319,#8974,#8975);
#7626=AXIS2_PLACEMENT_3D('',#21327,#8977,#8978);
#7627=AXIS2_PLACEMENT_3D('',#21334,#8979,#8980);
#7628=AXIS2_PLACEMENT_3D('',#21343,#8981,#8982);
#7629=AXIS2_PLACEMENT_3D('',#21352,#8983,#8984);
#7630=AXIS2_PLACEMENT_3D('',#21361,#8985,#8986);
#7631=AXIS2_PLACEMENT_3D('',#21370,#8987,#8988);
#7632=AXIS2_PLACEMENT_3D('',#21378,#8989,#8990);
#7633=AXIS2_PLACEMENT_3D('',#21379,#8991,#8992);
#7634=AXIS2_PLACEMENT_3D('',#21381,#8993,#8994);
#7635=AXIS2_PLACEMENT_3D('',#21392,#8995,#8996);
#7636=AXIS2_PLACEMENT_3D('',#21395,#8997,#8998);
#7637=AXIS2_PLACEMENT_3D('',#21431,#8999,#9000);
#7638=AXIS2_PLACEMENT_3D('',#21433,#9001,#9002);
#7639=AXIS2_PLACEMENT_3D('',#21445,#9003,#9004);
#7640=AXIS2_PLACEMENT_3D('',#21447,#9005,#9006);
#7641=AXIS2_PLACEMENT_3D('',#21458,#9007,#9008);
#7642=AXIS2_PLACEMENT_3D('',#21461,#9009,#9010);
#7643=AXIS2_PLACEMENT_3D('',#21497,#9011,#9012);
#7644=AXIS2_PLACEMENT_3D('',#21499,#9013,#9014);
#7645=AXIS2_PLACEMENT_3D('',#21511,#9015,#9016);
#7646=AXIS2_PLACEMENT_3D('',#21513,#9017,#9018);
#7647=AXIS2_PLACEMENT_3D('',#21524,#9019,#9020);
#7648=AXIS2_PLACEMENT_3D('',#21527,#9021,#9022);
#7649=AXIS2_PLACEMENT_3D('',#21563,#9023,#9024);
#7650=AXIS2_PLACEMENT_3D('',#21565,#9025,#9026);
#7651=AXIS2_PLACEMENT_3D('',#21577,#9027,#9028);
#7652=AXIS2_PLACEMENT_3D('',#21579,#9029,#9030);
#7653=AXIS2_PLACEMENT_3D('',#21590,#9031,#9032);
#7654=AXIS2_PLACEMENT_3D('',#21593,#9033,#9034);
#7655=AXIS2_PLACEMENT_3D('',#21635,#9035,#9036);
#7656=AXIS2_PLACEMENT_3D('',#21637,#9037,#9038);
#7657=AXIS2_PLACEMENT_3D('',#21649,#9039,#9040);
#7658=AXIS2_PLACEMENT_3D('',#21651,#9041,#9042);
#7659=AXIS2_PLACEMENT_3D('',#21662,#9043,#9044);
#7660=AXIS2_PLACEMENT_3D('',#21665,#9045,#9046);
#7661=AXIS2_PLACEMENT_3D('',#21701,#9047,#9048);
#7662=AXIS2_PLACEMENT_3D('',#21703,#9049,#9050);
#7663=AXIS2_PLACEMENT_3D('',#21715,#9051,#9052);
#7664=AXIS2_PLACEMENT_3D('',#21717,#9053,#9054);
#7665=AXIS2_PLACEMENT_3D('',#21728,#9055,#9056);
#7666=AXIS2_PLACEMENT_3D('',#21731,#9057,#9058);
#7667=AXIS2_PLACEMENT_3D('',#21767,#9059,#9060);
#7668=AXIS2_PLACEMENT_3D('',#21769,#9061,#9062);
#7669=AXIS2_PLACEMENT_3D('',#21781,#9063,#9064);
#7670=AXIS2_PLACEMENT_3D('',#21783,#9065,#9066);
#7671=AXIS2_PLACEMENT_3D('',#21794,#9067,#9068);
#7672=AXIS2_PLACEMENT_3D('',#21797,#9069,#9070);
#7673=AXIS2_PLACEMENT_3D('',#21833,#9071,#9072);
#7674=AXIS2_PLACEMENT_3D('',#21835,#9073,#9074);
#7675=AXIS2_PLACEMENT_3D('',#21847,#9075,#9076);
#7676=AXIS2_PLACEMENT_3D('',#21849,#9077,#9078);
#7677=AXIS2_PLACEMENT_3D('',#21860,#9079,#9080);
#7678=AXIS2_PLACEMENT_3D('',#21863,#9081,#9082);
#7679=AXIS2_PLACEMENT_3D('',#21899,#9083,#9084);
#7680=AXIS2_PLACEMENT_3D('',#21901,#9085,#9086);
#7681=AXIS2_PLACEMENT_3D('',#21909,#9087,#9088);
#7682=AXIS2_PLACEMENT_3D('',#21912,#9090,#9091);
#7683=AXIS2_PLACEMENT_3D('',#21913,#9092,#9093);
#7684=AXIS2_PLACEMENT_3D('',#21925,#9094,#9095);
#7685=AXIS2_PLACEMENT_3D('',#21927,#9096,#9097);
#7686=AXIS2_PLACEMENT_3D('',#21930,#9099,#9100);
#7687=AXIS2_PLACEMENT_3D('',#21938,#9101,#9102);
#7688=AXIS2_PLACEMENT_3D('',#21939,#9103,#9104);
#7689=AXIS2_PLACEMENT_3D('',#21950,#9105,#9106);
#7690=AXIS2_PLACEMENT_3D('',#21953,#9107,#9108);
#7691=AXIS2_PLACEMENT_3D('',#21975,#9109,#9110);
#7692=AXIS2_PLACEMENT_3D('',#21976,#9111,#9112);
#7693=AXIS2_PLACEMENT_3D('',#21978,#9113,#9114);
#7694=AXIS2_PLACEMENT_3D('',#21979,#9115,#9116);
#7695=AXIS2_PLACEMENT_3D('',#21981,#9117,#9118);
#7696=AXIS2_PLACEMENT_3D('',#21983,#9120,#9121);
#7697=AXIS2_PLACEMENT_3D('',#21985,#9122,#9123);
#7698=AXIS2_PLACEMENT_3D('',#21987,#9125,#9126);
#7699=AXIS2_PLACEMENT_3D('',#21989,#9127,#9128);
#7700=AXIS2_PLACEMENT_3D('',#21991,#9130,#9131);
#7701=AXIS2_PLACEMENT_3D('',#21993,#9132,#9133);
#7702=AXIS2_PLACEMENT_3D('',#21994,#9134,#9135);
#7703=AXIS2_PLACEMENT_3D('',#21996,#9137,#9138);
#7704=AXIS2_PLACEMENT_3D('',#21997,#9139,#9140);
#7705=AXIS2_PLACEMENT_3D('',#21999,#9141,#9142);
#7706=AXIS2_PLACEMENT_3D('',#22000,#9143,#9144);
#7707=AXIS2_PLACEMENT_3D('',#22003,#9146,#9147);
#7708=AXIS2_PLACEMENT_3D('',#22004,#9148,#9149);
#7709=AXIS2_PLACEMENT_3D('',#22007,#9151,#9152);
#7710=AXIS2_PLACEMENT_3D('',#22008,#9153,#9154);
#7711=AXIS2_PLACEMENT_3D('',#22011,#9156,#9157);
#7712=AXIS2_PLACEMENT_3D('',#22012,#9158,#9159);
#8931=DIRECTION('axis',(0.,0.,1.));
#8932=DIRECTION('refdir',(1.,0.,0.));
#8933=DIRECTION('center_axis',(0.,0.587785252292474,0.809016994374947));
#8934=DIRECTION('ref_axis',(1.,0.,0.));
#8935=DIRECTION('center_axis',(0.,-0.809016994374947,0.587785252292473));
#8936=DIRECTION('ref_axis',(-1.,0.,0.));
#8937=DIRECTION('center_axis',(1.,0.,0.));
#8938=DIRECTION('ref_axis',(0.,1.,0.));
#8939=DIRECTION('center_axis',(1.,0.,0.));
#8940=DIRECTION('ref_axis',(0.,0.,-1.));
#8941=DIRECTION('',(-0.53037253640964,0.847764691776206,1.03821231621387E-16));
#8942=DIRECTION('center_axis',(1.,0.,0.));
#8943=DIRECTION('ref_axis',(0.,0.,-1.));
#8944=DIRECTION('center_axis',(1.,0.,0.));
#8945=DIRECTION('ref_axis',(0.,0.,-1.));
#8946=DIRECTION('center_axis',(1.,0.,0.));
#8947=DIRECTION('ref_axis',(0.,0.,-1.));
#8948=DIRECTION('center_axis',(1.,0.,0.));
#8949=DIRECTION('ref_axis',(0.,0.,-1.));
#8950=DIRECTION('center_axis',(1.,0.,0.));
#8951=DIRECTION('ref_axis',(0.,0.,-1.));
#8952=DIRECTION('center_axis',(1.,0.,0.));
#8953=DIRECTION('ref_axis',(0.,0.,-1.));
#8954=DIRECTION('center_axis',(1.,0.,0.));
#8955=DIRECTION('ref_axis',(0.,0.,-1.));
#8956=DIRECTION('center_axis',(1.,0.,0.));
#8957=DIRECTION('ref_axis',(0.,0.,-1.));
#8958=DIRECTION('center_axis',(1.,0.,0.));
#8959=DIRECTION('ref_axis',(0.,0.,-1.));
#8960=DIRECTION('center_axis',(1.,0.,0.));
#8961=DIRECTION('ref_axis',(0.,0.,-1.));
#8962=DIRECTION('center_axis',(1.,0.,0.));
#8963=DIRECTION('ref_axis',(0.,0.,-1.));
#8964=DIRECTION('center_axis',(1.,0.,0.));
#8965=DIRECTION('ref_axis',(0.,0.,-1.));
#8966=DIRECTION('center_axis',(1.,0.,0.));
#8967=DIRECTION('ref_axis',(0.,1.,0.));
#8968=DIRECTION('center_axis',(1.,0.,0.));
#8969=DIRECTION('ref_axis',(0.,0.,-1.));
#8970=DIRECTION('center_axis',(1.,0.,0.));
#8971=DIRECTION('ref_axis',(0.,0.,-1.));
#8972=DIRECTION('center_axis',(1.,0.,0.));
#8973=DIRECTION('ref_axis',(0.,0.,-1.));
#8974=DIRECTION('center_axis',(1.,0.,0.));
#8975=DIRECTION('ref_axis',(0.,0.,-1.));
#8976=DIRECTION('',(-1.,0.,0.));
#8977=DIRECTION('center_axis',(1.,0.,0.));
#8978=DIRECTION('ref_axis',(0.,0.,-1.));
#8979=DIRECTION('center_axis',(1.,0.,0.));
#8980=DIRECTION('ref_axis',(0.,0.,-1.));
#8981=DIRECTION('center_axis',(1.,0.,0.));
#8982=DIRECTION('ref_axis',(0.,0.,-1.));
#8983=DIRECTION('center_axis',(1.,0.,0.));
#8984=DIRECTION('ref_axis',(0.,0.,-1.));
#8985=DIRECTION('center_axis',(1.,0.,0.));
#8986=DIRECTION('ref_axis',(0.,0.,-1.));
#8987=DIRECTION('center_axis',(1.,0.,0.));
#8988=DIRECTION('ref_axis',(0.,0.,-1.));
#8989=DIRECTION('center_axis',(1.,0.,0.));
#8990=DIRECTION('ref_axis',(0.,0.,-1.));
#8991=DIRECTION('center_axis',(1.,0.,0.));
#8992=DIRECTION('ref_axis',(0.,0.,-1.));
#8993=DIRECTION('center_axis',(1.,0.,0.));
#8994=DIRECTION('ref_axis',(0.,0.,-1.));
#8995=DIRECTION('center_axis',(0.,0.951056516295154,0.309016994374948));
#8996=DIRECTION('ref_axis',(1.,0.,0.));
#8997=DIRECTION('center_axis',(0.,-0.309016994374947,0.951056516295154));
#8998=DIRECTION('ref_axis',(-1.,0.,0.));
#8999=DIRECTION('center_axis',(1.,0.,0.));
#9000=DIRECTION('ref_axis',(0.,0.,-1.));
#9001=DIRECTION('center_axis',(1.,0.,0.));
#9002=DIRECTION('ref_axis',(0.,0.,-1.));
#9003=DIRECTION('center_axis',(1.,0.,0.));
#9004=DIRECTION('ref_axis',(0.,0.,-1.));
#9005=DIRECTION('center_axis',(1.,0.,0.));
#9006=DIRECTION('ref_axis',(0.,0.,-1.));
#9007=DIRECTION('center_axis',(0.,0.951056516295154,-0.309016994374948));
#9008=DIRECTION('ref_axis',(1.,0.,0.));
#9009=DIRECTION('center_axis',(0.,0.309016994374948,0.951056516295154));
#9010=DIRECTION('ref_axis',(-1.,0.,0.));
#9011=DIRECTION('center_axis',(1.,0.,0.));
#9012=DIRECTION('ref_axis',(0.,0.,-1.));
#9013=DIRECTION('center_axis',(1.,0.,0.));
#9014=DIRECTION('ref_axis',(0.,0.,-1.));
#9015=DIRECTION('center_axis',(1.,0.,0.));
#9016=DIRECTION('ref_axis',(0.,0.,-1.));
#9017=DIRECTION('center_axis',(1.,0.,0.));
#9018=DIRECTION('ref_axis',(0.,0.,-1.));
#9019=DIRECTION('center_axis',(0.,0.587785252292473,-0.809016994374947));
#9020=DIRECTION('ref_axis',(1.,0.,0.));
#9021=DIRECTION('center_axis',(0.,0.809016994374948,0.587785252292473));
#9022=DIRECTION('ref_axis',(-1.,0.,0.));
#9023=DIRECTION('center_axis',(1.,0.,0.));
#9024=DIRECTION('ref_axis',(0.,0.,-1.));
#9025=DIRECTION('center_axis',(1.,0.,0.));
#9026=DIRECTION('ref_axis',(0.,0.,-1.));
#9027=DIRECTION('center_axis',(1.,0.,0.));
#9028=DIRECTION('ref_axis',(0.,0.,-1.));
#9029=DIRECTION('center_axis',(1.,0.,0.));
#9030=DIRECTION('ref_axis',(0.,0.,-1.));
#9031=DIRECTION('center_axis',(0.,0.,-1.));
#9032=DIRECTION('ref_axis',(1.,0.,0.));
#9033=DIRECTION('center_axis',(0.,1.,-1.22464679914735E-16));
#9034=DIRECTION('ref_axis',(-1.,0.,0.));
#9035=DIRECTION('center_axis',(1.,0.,0.));
#9036=DIRECTION('ref_axis',(0.,0.,-1.));
#9037=DIRECTION('center_axis',(1.,0.,0.));
#9038=DIRECTION('ref_axis',(0.,0.,-1.));
#9039=DIRECTION('center_axis',(1.,0.,0.));
#9040=DIRECTION('ref_axis',(0.,0.,-1.));
#9041=DIRECTION('center_axis',(1.,0.,0.));
#9042=DIRECTION('ref_axis',(0.,0.,-1.));
#9043=DIRECTION('center_axis',(0.,-0.587785252292473,-0.809016994374948));
#9044=DIRECTION('ref_axis',(1.,0.,0.));
#9045=DIRECTION('center_axis',(0.,0.809016994374947,-0.587785252292473));
#9046=DIRECTION('ref_axis',(-1.,0.,0.));
#9047=DIRECTION('center_axis',(1.,0.,0.));
#9048=DIRECTION('ref_axis',(0.,0.,-1.));
#9049=DIRECTION('center_axis',(1.,0.,0.));
#9050=DIRECTION('ref_axis',(0.,0.,-1.));
#9051=DIRECTION('center_axis',(1.,0.,0.));
#9052=DIRECTION('ref_axis',(0.,0.,-1.));
#9053=DIRECTION('center_axis',(1.,0.,0.));
#9054=DIRECTION('ref_axis',(0.,0.,-1.));
#9055=DIRECTION('center_axis',(0.,-0.951056516295154,-0.309016994374948));
#9056=DIRECTION('ref_axis',(1.,0.,0.));
#9057=DIRECTION('center_axis',(0.,0.309016994374947,-0.951056516295154));
#9058=DIRECTION('ref_axis',(-1.,0.,0.));
#9059=DIRECTION('center_axis',(1.,0.,0.));
#9060=DIRECTION('ref_axis',(0.,-1.22464679914735E-16,1.));
#9061=DIRECTION('center_axis',(1.,0.,0.));
#9062=DIRECTION('ref_axis',(0.,0.,-1.));
#9063=DIRECTION('center_axis',(1.,0.,0.));
#9064=DIRECTION('ref_axis',(0.,-1.22464679914735E-16,1.));
#9065=DIRECTION('center_axis',(1.,0.,0.));
#9066=DIRECTION('ref_axis',(0.,0.,-1.));
#9067=DIRECTION('center_axis',(0.,-0.951056516295154,0.309016994374948));
#9068=DIRECTION('ref_axis',(1.,0.,0.));
#9069=DIRECTION('center_axis',(0.,-0.309016994374948,-0.951056516295154));
#9070=DIRECTION('ref_axis',(-1.,0.,0.));
#9071=DIRECTION('center_axis',(1.,0.,0.));
#9072=DIRECTION('ref_axis',(0.,0.,-1.));
#9073=DIRECTION('center_axis',(1.,0.,0.));
#9074=DIRECTION('ref_axis',(0.,0.,-1.));
#9075=DIRECTION('center_axis',(1.,0.,0.));
#9076=DIRECTION('ref_axis',(0.,0.,-1.));
#9077=DIRECTION('center_axis',(1.,0.,0.));
#9078=DIRECTION('ref_axis',(0.,0.,-1.));
#9079=DIRECTION('center_axis',(0.,-0.587785252292473,0.809016994374947));
#9080=DIRECTION('ref_axis',(1.,0.,0.));
#9081=DIRECTION('center_axis',(0.,-0.809016994374948,-0.587785252292473));
#9082=DIRECTION('ref_axis',(-1.,0.,0.));
#9083=DIRECTION('center_axis',(1.,0.,0.));
#9084=DIRECTION('ref_axis',(0.,1.,0.));
#9085=DIRECTION('center_axis',(1.,0.,0.));
#9086=DIRECTION('ref_axis',(0.,0.,-1.));
#9087=DIRECTION('center_axis',(1.,0.,0.));
#9088=DIRECTION('ref_axis',(0.,0.,-1.));
#9089=DIRECTION('',(-1.,0.,0.));
#9090=DIRECTION('center_axis',(1.,0.,0.));
#9091=DIRECTION('ref_axis',(0.,0.,-1.));
#9092=DIRECTION('center_axis',(1.,0.,0.));
#9093=DIRECTION('ref_axis',(0.,0.,-1.));
#9094=DIRECTION('center_axis',(1.,0.,0.));
#9095=DIRECTION('ref_axis',(0.,1.,0.));
#9096=DIRECTION('center_axis',(1.,0.,0.));
#9097=DIRECTION('ref_axis',(0.,0.,-1.));
#9098=DIRECTION('',(-1.,0.,0.));
#9099=DIRECTION('center_axis',(1.,0.,0.));
#9100=DIRECTION('ref_axis',(0.,0.,-1.));
#9101=DIRECTION('center_axis',(1.,0.,0.));
#9102=DIRECTION('ref_axis',(0.,0.,-1.));
#9103=DIRECTION('center_axis',(1.,0.,0.));
#9104=DIRECTION('ref_axis',(0.,0.,-1.));
#9105=DIRECTION('center_axis',(0.,0.,1.));
#9106=DIRECTION('ref_axis',(1.,0.,0.));
#9107=DIRECTION('center_axis',(0.,-1.,0.));
#9108=DIRECTION('ref_axis',(-1.,0.,0.));
#9109=DIRECTION('center_axis',(1.,0.,0.));
#9110=DIRECTION('ref_axis',(0.,0.,-1.));
#9111=DIRECTION('center_axis',(-1.,0.,0.));
#9112=DIRECTION('ref_axis',(0.,0.,1.));
#9113=DIRECTION('center_axis',(1.,0.,0.));
#9114=DIRECTION('ref_axis',(0.,0.,-1.));
#9115=DIRECTION('center_axis',(1.,0.,0.));
#9116=DIRECTION('ref_axis',(0.,1.,0.));
#9117=DIRECTION('center_axis',(1.,0.,0.));
#9118=DIRECTION('ref_axis',(0.,0.,-1.));
#9119=DIRECTION('',(-0.707106781186547,0.707106781186548,8.65956056235494E-17));
#9120=DIRECTION('center_axis',(1.,0.,0.));
#9121=DIRECTION('ref_axis',(0.,1.,0.));
#9122=DIRECTION('center_axis',(1.,0.,0.));
#9123=DIRECTION('ref_axis',(0.,0.,-1.));
#9124=DIRECTION('',(-1.,0.,0.));
#9125=DIRECTION('center_axis',(-1.,0.,0.));
#9126=DIRECTION('ref_axis',(0.,1.,0.));
#9127=DIRECTION('center_axis',(1.,0.,0.));
#9128=DIRECTION('ref_axis',(0.,0.,-1.));
#9129=DIRECTION('',(-0.707106781186548,-0.707106781186548,-8.65956056235493E-17));
#9130=DIRECTION('center_axis',(1.,0.,0.));
#9131=DIRECTION('ref_axis',(0.,0.,-1.));
#9132=DIRECTION('center_axis',(1.,0.,0.));
#9133=DIRECTION('ref_axis',(0.,0.,-1.));
#9134=DIRECTION('center_axis',(1.,0.,0.));
#9135=DIRECTION('ref_axis',(0.,1.,0.));
#9136=DIRECTION('',(-1.,0.,0.));
#9137=DIRECTION('center_axis',(1.,0.,0.));
#9138=DIRECTION('ref_axis',(0.,0.,-1.));
#9139=DIRECTION('center_axis',(1.,0.,0.));
#9140=DIRECTION('ref_axis',(0.,0.,-1.));
#9141=DIRECTION('center_axis',(1.,0.,0.));
#9142=DIRECTION('ref_axis',(0.,0.,-1.));
#9143=DIRECTION('center_axis',(1.,0.,0.));
#9144=DIRECTION('ref_axis',(0.,1.,0.));
#9145=DIRECTION('',(-0.707106781186548,0.707106781186548,8.65956056235493E-17));
#9146=DIRECTION('center_axis',(1.,0.,0.));
#9147=DIRECTION('ref_axis',(0.,0.,-1.));
#9148=DIRECTION('center_axis',(1.,0.,0.));
#9149=DIRECTION('ref_axis',(0.,1.,0.));
#9150=DIRECTION('',(-1.,0.,0.));
#9151=DIRECTION('center_axis',(1.,0.,0.));
#9152=DIRECTION('ref_axis',(0.,0.,-1.));
#9153=DIRECTION('center_axis',(-1.,0.,0.));
#9154=DIRECTION('ref_axis',(0.,1.,0.));
#9155=DIRECTION('',(-0.707106781186547,-0.707106781186548,-8.65956056235494E-17));
#9156=DIRECTION('center_axis',(1.,0.,0.));
#9157=DIRECTION('ref_axis',(0.,0.,-1.));
#9158=DIRECTION('center_axis',(-1.,0.,0.));
#9159=DIRECTION('ref_axis',(0.,0.,1.));
#21108=CARTESIAN_POINT('',(0.,0.,0.));
#21109=CARTESIAN_POINT('Origin',(4.,8.09016994374947,-5.87785252292473));
#21110=CARTESIAN_POINT('',(4.,9.48983357577093,-3.95138080506939));
#21111=CARTESIAN_POINT('',(4.,6.69050631172802,-7.80432424078008));
#21112=CARTESIAN_POINT('Origin',(4.,8.09016994374947,-5.87785252292473));
#21113=CARTESIAN_POINT('',(2.36305161962877,9.25963747468151,-7.15186086536042));
#21114=CARTESIAN_POINT('',(2.36305161962877,9.66320922106503,-6.59639201002517));
#21115=CARTESIAN_POINT('Ctrl Pts',(2.36305161962876,9.25963747468151,-7.15186086536042));
#21116=CARTESIAN_POINT('Ctrl Pts',(2.34215062955512,9.33091437868292,-7.05957742979088));
#21117=CARTESIAN_POINT('Ctrl Pts',(2.33256137669178,9.40089182481285,-6.96601137146006));
#21118=CARTESIAN_POINT('Ctrl Pts',(2.33256137669178,9.53010584356091,-6.78816353218381));
#21119=CARTESIAN_POINT('Ctrl Pts',(2.34215062955512,9.59746823296338,-6.69269752392735));
#21120=CARTESIAN_POINT('Ctrl Pts',(2.36305161962876,9.66320922106503,-6.59639201002516));
#21121=CARTESIAN_POINT('',(5.63694838037123,9.25963747468151,-7.15186086536042));
#21122=CARTESIAN_POINT('Ctrl Pts',(5.63694838037123,9.25963747468149,-7.15186086536043));
#21123=CARTESIAN_POINT('Ctrl Pts',(5.43435664662035,9.41577612470672,-7.26884057730417));
#21124=CARTESIAN_POINT('Ctrl Pts',(5.15858882449494,9.55944543027121,-7.37642824958397));
#21125=CARTESIAN_POINT('Ctrl Pts',(4.63402456511048,9.73338541206091,-7.5066654368745));
#21126=CARTESIAN_POINT('Ctrl Pts',(4.2912458937239,9.7879741784414,-7.54752684540867));
#21127=CARTESIAN_POINT('Ctrl Pts',(4.,9.7879741784414,-7.54752684540867));
#21128=CARTESIAN_POINT('Ctrl Pts',(3.7087541062761,9.7879741784414,-7.54752684540867));
#21129=CARTESIAN_POINT('Ctrl Pts',(3.36597543488952,9.73338541206091,-7.5066654368745));
#21130=CARTESIAN_POINT('Ctrl Pts',(2.84141117550506,9.55944543027121,-7.37642824958397));
#21131=CARTESIAN_POINT('Ctrl Pts',(2.56564335337965,9.41577612470672,-7.26884057730417));
#21132=CARTESIAN_POINT('Ctrl Pts',(2.36305161962877,9.25963747468149,-7.15186086536043));
#21133=CARTESIAN_POINT('',(5.63694838037123,9.66320922106503,-6.59639201002517));
#21134=CARTESIAN_POINT('Ctrl Pts',(5.63694838037123,9.66320922106503,-6.59639201002517));
#21135=CARTESIAN_POINT('Ctrl Pts',(5.64480038182766,9.6077764900278,-6.69985819864571));
#21136=CARTESIAN_POINT('Ctrl Pts',(5.64846349832042,9.5458342503805,-6.79782963077036));
#21137=CARTESIAN_POINT('Ctrl Pts',(5.64846349832042,9.41494517586244,-6.97798298652422));
#21138=CARTESIAN_POINT('Ctrl Pts',(5.64480038182766,9.34091001165019,-7.06716839466448));
#21139=CARTESIAN_POINT('Ctrl Pts',(5.63694838037123,9.25963747468151,-7.15186086536042));
#21140=CARTESIAN_POINT('Ctrl Pts',(2.36305161962877,9.66320922106504,-6.59639201002515));
#21141=CARTESIAN_POINT('Ctrl Pts',(2.56564335337965,9.82271303472001,-6.70873997158947));
#21142=CARTESIAN_POINT('Ctrl Pts',(2.84141117550506,9.96943124850423,-6.81213118171848));
#21143=CARTESIAN_POINT('Ctrl Pts',(3.36597543488952,10.1470445845151,-6.93731243067146));
#21144=CARTESIAN_POINT('Ctrl Pts',(3.7087541062761,10.2027749498801,-6.97660256300298));
#21145=CARTESIAN_POINT('Ctrl Pts',(4.,10.2027749498801,-6.97660256300298));
#21146=CARTESIAN_POINT('Ctrl Pts',(4.2912458937239,10.2027749498801,-6.97660256300298));
#21147=CARTESIAN_POINT('Ctrl Pts',(4.63402456511048,10.1470445845151,-6.93731243067146));
#21148=CARTESIAN_POINT('Ctrl Pts',(5.15858882449494,9.96943124850423,-6.81213118171848));
#21149=CARTESIAN_POINT('Ctrl Pts',(5.43435664662035,9.82271303472001,-6.70873997158947));
#21150=CARTESIAN_POINT('Ctrl Pts',(5.63694838037123,9.66320922106504,-6.59639201002515));
#21151=CARTESIAN_POINT('',(5.63694838037123,6.54081691696393,-5.10957082921438));
#21152=CARTESIAN_POINT('',(5.63694838037123,6.88071421703296,-4.64174233058239));
#21153=CARTESIAN_POINT('Ctrl Pts',(5.63694838037124,6.54081691696393,-5.10957082921438));
#21154=CARTESIAN_POINT('Ctrl Pts',(5.6577376463315,6.60095637772735,-5.03258565462996));
#21155=CARTESIAN_POINT('Ctrl Pts',(5.66743862330822,6.66027285287123,-4.95372427854694));
#21156=CARTESIAN_POINT('Ctrl Pts',(5.66743862330822,6.7694092537529,-4.80351090950812));
#21157=CARTESIAN_POINT('Ctrl Pts',(5.6577376463315,6.82608108049478,-4.72272808388943));
#21158=CARTESIAN_POINT('Ctrl Pts',(5.63694838037124,6.88071421703297,-4.64174233058239));
#21159=CARTESIAN_POINT('',(2.36305161962877,6.54081691696392,-5.10957082921439));
#21160=CARTESIAN_POINT('Ctrl Pts',(2.36305161962877,6.54081691696392,-5.10957082921439));
#21161=CARTESIAN_POINT('Ctrl Pts',(2.56564497161068,6.38499222767917,-4.99215633639486));
#21162=CARTESIAN_POINT('Ctrl Pts',(2.8414185613243,6.24167414543094,-4.88407927525699));
#21163=CARTESIAN_POINT('Ctrl Pts',(3.36598484931781,6.06819253427498,-4.75321678286295));
#21164=CARTESIAN_POINT('Ctrl Pts',(3.70875810561651,6.0137647807275,-4.71213679365121));
#21165=CARTESIAN_POINT('Ctrl Pts',(4.29124189438349,6.0137647807275,-4.71213679365121));
#21166=CARTESIAN_POINT('Ctrl Pts',(4.6340151506822,6.06819253427498,-4.75321678286295));
#21167=CARTESIAN_POINT('Ctrl Pts',(5.1585814386757,6.24167414543094,-4.88407927525699));
#21168=CARTESIAN_POINT('Ctrl Pts',(5.43435502838932,6.38499222767917,-4.99215633639486));
#21169=CARTESIAN_POINT('Ctrl Pts',(5.63694838037123,6.54081691696391,-5.10957082921439));
#21170=CARTESIAN_POINT('',(2.36305161962877,6.88071421703297,-4.64174233058238));
#21171=CARTESIAN_POINT('Ctrl Pts',(2.36305161962877,6.88071421703297,-4.64174233058238));
#21172=CARTESIAN_POINT('Ctrl Pts',(2.3422623536685,6.82608108049479,-4.72272808388942));
#21173=CARTESIAN_POINT('Ctrl Pts',(2.33256137669178,6.7694092537529,-4.80351090950811));
#21174=CARTESIAN_POINT('Ctrl Pts',(2.33256137669178,6.66027285287122,-4.95372427854695));
#21175=CARTESIAN_POINT('Ctrl Pts',(2.3422623536685,6.60095637772735,-5.03258565462997));
#21176=CARTESIAN_POINT('Ctrl Pts',(2.36305161962877,6.54081691696392,-5.10957082921439));
#21177=CARTESIAN_POINT('Ctrl Pts',(5.63694838037123,6.88071421703298,-4.64174233058237));
#21178=CARTESIAN_POINT('Ctrl Pts',(5.43435502838932,6.72089392139729,-4.5298273181056));
#21179=CARTESIAN_POINT('Ctrl Pts',(5.1585814386757,6.57381880512416,-4.4269213706742));
#21180=CARTESIAN_POINT('Ctrl Pts',(4.6340151506822,6.39575241293544,-4.30236928800296));
#21181=CARTESIAN_POINT('Ctrl Pts',(4.29124189438349,6.33986392069446,-4.2632998331195));
#21182=CARTESIAN_POINT('Ctrl Pts',(3.70875810561651,6.33986392069446,-4.2632998331195));
#21183=CARTESIAN_POINT('Ctrl Pts',(3.36598484931781,6.39575241293544,-4.30236928800296));
#21184=CARTESIAN_POINT('Ctrl Pts',(2.8414185613243,6.57381880512416,-4.4269213706742));
#21185=CARTESIAN_POINT('Ctrl Pts',(2.56564497161068,6.72089392139729,-4.5298273181056));
#21186=CARTESIAN_POINT('Ctrl Pts',(2.36305161962877,6.88071421703298,-4.64174233058237));
#21187=CARTESIAN_POINT('Origin',(5.91847419018562,0.,0.));
#21188=CARTESIAN_POINT('',(6.2,-12.6,-1.54305496692567E-15));
#21189=CARTESIAN_POINT('Origin',(6.2,0.,0.));
#21190=CARTESIAN_POINT('',(5.64846349832042,-11.7184061386079,-5.83505075665543E-17));
#21191=CARTESIAN_POINT('',(5.91847419018562,-12.15,-1.48794586096403E-15));
#21192=CARTESIAN_POINT('',(5.63694838037123,-11.694962421875,0.343298632289184));
#21193=CARTESIAN_POINT('Ctrl Pts',(5.64846349832042,-11.7184061386079,1.31838984174237E-15));
#21194=CARTESIAN_POINT('Ctrl Pts',(5.64846349832042,-11.7184061386079,0.11134089704324));
#21195=CARTESIAN_POINT('Ctrl Pts',(5.64480038182766,-11.7109323002033,0.227010185553986));
#21196=CARTESIAN_POINT('Ctrl Pts',(5.63694838037123,-11.694962421875,0.343298632289185));
#21197=CARTESIAN_POINT('',(5.63694838037123,-9.66320922106502,6.59639201002516));
#21198=CARTESIAN_POINT('Origin',(5.63694838037123,0.,0.));
#21199=CARTESIAN_POINT('',(5.63694838037123,-9.25963747468151,7.15186086536042));
#21200=CARTESIAN_POINT('Ctrl Pts',(5.63694838037123,-9.66320922106503,6.59639201002517));
#21201=CARTESIAN_POINT('Ctrl Pts',(5.64480038182766,-9.6077764900278,6.69985819864571));
#21202=CARTESIAN_POINT('Ctrl Pts',(5.64846349832042,-9.5458342503805,6.79782963077036));
#21203=CARTESIAN_POINT('Ctrl Pts',(5.64846349832042,-9.41494517586244,6.97798298652422));
#21204=CARTESIAN_POINT('Ctrl Pts',(5.64480038182766,-9.34091001165019,7.06716839466448));
#21205=CARTESIAN_POINT('Ctrl Pts',(5.63694838037123,-9.25963747468151,7.15186086536042));
#21206=CARTESIAN_POINT('',(5.63694838037123,-3.94043853820961,11.0164851076281));
#21207=CARTESIAN_POINT('Origin',(5.63694838037123,0.,0.));
#21208=CARTESIAN_POINT('',(5.63694838037123,-3.28744573566193,11.2286553306742));
#21209=CARTESIAN_POINT('Ctrl Pts',(5.63694838037123,-3.94043853820961,11.0164851076281));
#21210=CARTESIAN_POINT('Ctrl Pts',(5.64480038182766,-3.83477661697381,11.0676084707674));
#21211=CARTESIAN_POINT('Ctrl Pts',(5.64846349832042,-3.72707812948065,11.1104602893608));
#21212=CARTESIAN_POINT('Ctrl Pts',(5.64846349832042,-3.51529515815442,11.1792727480714));
#21213=CARTESIAN_POINT('Ctrl Pts',(5.64480038182766,-3.40297758450084,11.2079084812322));
#21214=CARTESIAN_POINT('Ctrl Pts',(5.63694838037123,-3.28744573566193,11.2286553306742));
#21215=CARTESIAN_POINT('',(5.63694838037123,3.28744573566193,11.2286553306742));
#21216=CARTESIAN_POINT('Origin',(5.63694838037123,0.,0.));
#21217=CARTESIAN_POINT('',(5.63694838037123,3.94043853820961,11.0164851076281));
#21218=CARTESIAN_POINT('Ctrl Pts',(5.63694838037123,3.28744573566193,11.2286553306742));
#21219=CARTESIAN_POINT('Ctrl Pts',(5.64480038182766,3.40297758450084,11.2079084812322));
#21220=CARTESIAN_POINT('Ctrl Pts',(5.64846349832042,3.51529515815442,11.1792727480715));
#21221=CARTESIAN_POINT('Ctrl Pts',(5.64846349832042,3.72707812948066,11.1104602893608));
#21222=CARTESIAN_POINT('Ctrl Pts',(5.64480038182766,3.83477661697381,11.0676084707674));
#21223=CARTESIAN_POINT('Ctrl Pts',(5.63694838037123,3.94043853820961,11.0164851076281));
#21224=CARTESIAN_POINT('',(5.63694838037123,9.25963747468151,7.15186086536041));
#21225=CARTESIAN_POINT('Origin',(5.63694838037123,0.,0.));
#21226=CARTESIAN_POINT('',(5.63694838037123,9.66320922106503,6.59639201002516));
#21227=CARTESIAN_POINT('Ctrl Pts',(5.63694838037123,9.25963747468151,7.15186086536041));
#21228=CARTESIAN_POINT('Ctrl Pts',(5.64480038182766,9.34091001165019,7.06716839466447));
#21229=CARTESIAN_POINT('Ctrl Pts',(5.64846349832042,9.41494517586244,6.97798298652422));
#21230=CARTESIAN_POINT('Ctrl Pts',(5.64846349832042,9.5458342503805,6.79782963077036));
#21231=CARTESIAN_POINT('Ctrl Pts',(5.64480038182766,9.6077764900278,6.69985819864571));
#21232=CARTESIAN_POINT('Ctrl Pts',(5.63694838037123,9.66320922106503,6.59639201002516));
#21233=CARTESIAN_POINT('',(5.63694838037123,11.694962421875,0.343298632289183));
#21234=CARTESIAN_POINT('Origin',(5.63694838037123,0.,0.));
#21235=CARTESIAN_POINT('',(5.63694838037123,11.694962421875,-0.343298632289183));
#21236=CARTESIAN_POINT('Ctrl Pts',(5.63694838037123,11.694962421875,0.343298632289183));
#21237=CARTESIAN_POINT('Ctrl Pts',(5.64480038182766,11.7109323002033,0.227010185553984));
#21238=CARTESIAN_POINT('Ctrl Pts',(5.64846349832042,11.7184061386079,0.111340897043238));
#21239=CARTESIAN_POINT('Ctrl Pts',(5.64846349832042,11.7184061386079,-0.111340897043237));
#21240=CARTESIAN_POINT('Ctrl Pts',(5.64480038182766,11.7109323002033,-0.227010185553985));
#21241=CARTESIAN_POINT('Ctrl Pts',(5.63694838037123,11.694962421875,-0.343298632289183));
#21242=CARTESIAN_POINT('Origin',(5.63694838037123,0.,0.));
#21243=CARTESIAN_POINT('',(5.63694838037123,3.94043853820961,-11.0164851076281));
#21244=CARTESIAN_POINT('Origin',(5.63694838037123,0.,0.));
#21245=CARTESIAN_POINT('',(5.63694838037123,3.28744573566193,-11.2286553306742));
#21246=CARTESIAN_POINT('Ctrl Pts',(5.63694838037123,3.94043853820961,-11.0164851076281));
#21247=CARTESIAN_POINT('Ctrl Pts',(5.64480038182766,3.83477661697381,-11.0676084707674));
#21248=CARTESIAN_POINT('Ctrl Pts',(5.64846349832042,3.72707812948065,-11.1104602893608));
#21249=CARTESIAN_POINT('Ctrl Pts',(5.64846349832042,3.51529515815441,-11.1792727480715));
#21250=CARTESIAN_POINT('Ctrl Pts',(5.64480038182766,3.40297758450083,-11.2079084812322));
#21251=CARTESIAN_POINT('Ctrl Pts',(5.63694838037123,3.28744573566193,-11.2286553306742));
#21252=CARTESIAN_POINT('',(5.63694838037123,-3.28744573566193,-11.2286553306742));
#21253=CARTESIAN_POINT('Origin',(5.63694838037123,0.,0.));
#21254=CARTESIAN_POINT('',(5.63694838037123,-3.94043853820961,-11.0164851076281));
#21255=CARTESIAN_POINT('Ctrl Pts',(5.63694838037123,-3.28744573566193,-11.2286553306742));
#21256=CARTESIAN_POINT('Ctrl Pts',(5.64480038182766,-3.40297758450084,-11.2079084812322));
#21257=CARTESIAN_POINT('Ctrl Pts',(5.64846349832042,-3.51529515815442,-11.1792727480715));
#21258=CARTESIAN_POINT('Ctrl Pts',(5.64846349832042,-3.72707812948065,-11.1104602893608));
#21259=CARTESIAN_POINT('Ctrl Pts',(5.64480038182766,-3.83477661697381,-11.0676084707674));
#21260=CARTESIAN_POINT('Ctrl Pts',(5.63694838037123,-3.94043853820961,-11.0164851076281));
#21261=CARTESIAN_POINT('',(5.63694838037123,-9.25963747468151,-7.15186086536041));
#21262=CARTESIAN_POINT('Origin',(5.63694838037123,0.,0.));
#21263=CARTESIAN_POINT('',(5.63694838037123,-9.66320922106503,-6.59639201002516));
#21264=CARTESIAN_POINT('Ctrl Pts',(5.63694838037123,-9.25963747468151,-7.15186086536042));
#21265=CARTESIAN_POINT('Ctrl Pts',(5.64480038182766,-9.34091001165019,-7.06716839466447));
#21266=CARTESIAN_POINT('Ctrl Pts',(5.64846349832042,-9.41494517586245,-6.97798298652421));
#21267=CARTESIAN_POINT('Ctrl Pts',(5.64846349832042,-9.54583425038051,-6.79782963077034));
#21268=CARTESIAN_POINT('Ctrl Pts',(5.64480038182766,-9.60777649002781,-6.6998581986457));
#21269=CARTESIAN_POINT('Ctrl Pts',(5.63694838037123,-9.66320922106503,-6.59639201002516));
#21270=CARTESIAN_POINT('',(5.63694838037123,-11.694962421875,-0.343298632289181));
#21271=CARTESIAN_POINT('Origin',(5.63694838037123,0.,0.));
#21272=CARTESIAN_POINT('Ctrl Pts',(5.63694838037123,-11.694962421875,-0.343298632289181));
#21273=CARTESIAN_POINT('Ctrl Pts',(5.64480038182766,-11.7109323002033,-0.227010185553983));
#21274=CARTESIAN_POINT('Ctrl Pts',(5.64846349832042,-11.7184061386079,-0.111340897043236));
#21275=CARTESIAN_POINT('Ctrl Pts',(5.64846349832042,-11.7184061386079,1.52655665885959E-15));
#21276=CARTESIAN_POINT('Origin',(4.,0.,0.));
#21277=CARTESIAN_POINT('',(2.36305161962877,3.94043853820961,-11.0164851076281));
#21278=CARTESIAN_POINT('Origin',(2.36305161962877,0.,0.));
#21279=CARTESIAN_POINT('Ctrl Pts',(2.36305161962877,3.94043853820962,-11.0164851076281));
#21280=CARTESIAN_POINT('Ctrl Pts',(2.56564335337965,4.00344335919148,-11.2011305071679));
#21281=CARTESIAN_POINT('Ctrl Pts',(2.84141117550506,4.06136905899675,-11.3710145555363));
#21282=CARTESIAN_POINT('Ctrl Pts',(3.36597543488952,4.13148157425907,-11.576686812834));
#21283=CARTESIAN_POINT('Ctrl Pts',(3.7087541062761,4.15347422659696,-11.6412306844678));
#21284=CARTESIAN_POINT('Ctrl Pts',(4.,4.15347422659696,-11.6412306844678));
#21285=CARTESIAN_POINT('Ctrl Pts',(4.2912458937239,4.15347422659696,-11.6412306844678));
#21286=CARTESIAN_POINT('Ctrl Pts',(4.63402456511048,4.13148157425907,-11.576686812834));
#21287=CARTESIAN_POINT('Ctrl Pts',(5.15858882449494,4.06136905899675,-11.3710145555363));
#21288=CARTESIAN_POINT('Ctrl Pts',(5.43435664662035,4.00344335919148,-11.2011305071679));
#21289=CARTESIAN_POINT('Ctrl Pts',(5.63694838037123,3.94043853820962,-11.0164851076281));
#21290=CARTESIAN_POINT('Origin',(1.18152580981438,0.,0.));
#21291=CARTESIAN_POINT('',(2.36305161962877,2.83826704815897,-7.79963077096185));
#21292=CARTESIAN_POINT('Origin',(2.36305161962877,0.,0.));
#21293=CARTESIAN_POINT('',(2.36305161962877,2.28830166396292,-7.97832535653345));
#21294=CARTESIAN_POINT('Ctrl Pts',(2.36305161962877,2.83826704815897,-7.79963077096185));
#21295=CARTESIAN_POINT('Ctrl Pts',(2.3422623536685,2.7464656808039,-7.83303706974588));
#21296=CARTESIAN_POINT('Ctrl Pts',(2.33256137669178,2.65313425633026,-7.86508088454567));
#21297=CARTESIAN_POINT('Ctrl Pts',(2.33256137669178,2.47654785029387,-7.92245728595388));
#21298=CARTESIAN_POINT('Ctrl Pts',(2.3422623536685,2.38220626001896,-7.95139213009729));
#21299=CARTESIAN_POINT('Ctrl Pts',(2.36305161962877,2.28830166396292,-7.97832535653345));
#21300=CARTESIAN_POINT('',(2.36305161962877,-2.28830166396292,-7.97832535653345));
#21301=CARTESIAN_POINT('Origin',(2.36305161962877,0.,0.));
#21302=CARTESIAN_POINT('',(2.36305161962877,-2.83826704815898,-7.79963077096185));
#21303=CARTESIAN_POINT('Ctrl Pts',(2.36305161962877,-2.28830166396292,-7.97832535653345));
#21304=CARTESIAN_POINT('Ctrl Pts',(2.3422623536685,-2.38220626001896,-7.95139213009729));
#21305=CARTESIAN_POINT('Ctrl Pts',(2.33256137669178,-2.47654785029387,-7.92245728595388));
#21306=CARTESIAN_POINT('Ctrl Pts',(2.33256137669178,-2.65313425633026,-7.86508088454567));
#21307=CARTESIAN_POINT('Ctrl Pts',(2.3422623536685,-2.7464656808039,-7.83303706974588));
#21308=CARTESIAN_POINT('Ctrl Pts',(2.36305161962877,-2.83826704815898,-7.79963077096185));
#21309=CARTESIAN_POINT('',(2.36305161962877,-6.54081691696392,-5.10957082921439));
#21310=CARTESIAN_POINT('Origin',(2.36305161962877,0.,0.));
#21311=CARTESIAN_POINT('',(2.36305161962877,-6.88071421703298,-4.64174233058237));
#21312=CARTESIAN_POINT('Ctrl Pts',(2.36305161962877,-6.54081691696392,-5.10957082921439));
#21313=CARTESIAN_POINT('Ctrl Pts',(2.3422623536685,-6.60095637772735,-5.03258565462997));
#21314=CARTESIAN_POINT('Ctrl Pts',(2.33256137669179,-6.66027285287123,-4.95372427854694));
#21315=CARTESIAN_POINT('Ctrl Pts',(2.33256137669178,-6.7694092537529,-4.80351090950811));
#21316=CARTESIAN_POINT('Ctrl Pts',(2.3422623536685,-6.82608108049479,-4.72272808388942));
#21317=CARTESIAN_POINT('Ctrl Pts',(2.36305161962877,-6.88071421703298,-4.64174233058237));
#21318=CARTESIAN_POINT('',(2.36305161962877,-8.294962421875,-0.289133913060418));
#21319=CARTESIAN_POINT('Origin',(2.36305161962877,0.,0.));
#21320=CARTESIAN_POINT('',(2.33256137669178,-8.3,-1.01563503836937E-15));
#21321=CARTESIAN_POINT('Ctrl Pts',(2.36305161962877,-8.294962421875,-0.289133913060418));
#21322=CARTESIAN_POINT('Ctrl Pts',(2.3422623536685,-8.29836551739928,-0.191502510389135));
#21323=CARTESIAN_POINT('Ctrl Pts',(2.33256137669178,-8.3,-0.0928369676306304));
#21324=CARTESIAN_POINT('Ctrl Pts',(2.33256137669178,-8.3,-1.01481323344643E-15));
#21325=CARTESIAN_POINT('',(0.,-8.3,-1.0164568432923E-15));
#21326=CARTESIAN_POINT('',(1.18152580981438,-8.3,-1.0164568432923E-15));
#21327=CARTESIAN_POINT('Origin',(0.,0.,0.));
#21328=CARTESIAN_POINT('',(2.36305161962877,-8.294962421875,0.28913391306042));
#21329=CARTESIAN_POINT('Ctrl Pts',(2.33256137669178,-8.3,-1.01481323344643E-15));
#21330=CARTESIAN_POINT('Ctrl Pts',(2.33256137669178,-8.3,0.0928369676306297));
#21331=CARTESIAN_POINT('Ctrl Pts',(2.3422623536685,-8.29836551739928,0.191502510389136));
#21332=CARTESIAN_POINT('Ctrl Pts',(2.36305161962877,-8.294962421875,0.28913391306042));
#21333=CARTESIAN_POINT('',(2.36305161962877,-6.88071421703297,4.64174233058237));
#21334=CARTESIAN_POINT('Origin',(2.36305161962877,0.,0.));
#21335=CARTESIAN_POINT('',(2.36305161962877,-6.54081691696392,5.10957082921439));
#21336=CARTESIAN_POINT('Ctrl Pts',(2.36305161962877,-6.88071421703297,4.64174233058237));
#21337=CARTESIAN_POINT('Ctrl Pts',(2.3422623536685,-6.82608108049479,4.72272808388942));
#21338=CARTESIAN_POINT('Ctrl Pts',(2.33256137669178,-6.7694092537529,4.80351090950811));
#21339=CARTESIAN_POINT('Ctrl Pts',(2.33256137669178,-6.66027285287123,4.95372427854694));
#21340=CARTESIAN_POINT('Ctrl Pts',(2.3422623536685,-6.60095637772735,5.03258565462997));
#21341=CARTESIAN_POINT('Ctrl Pts',(2.36305161962877,-6.54081691696392,5.10957082921439));
#21342=CARTESIAN_POINT('',(2.36305161962877,-2.83826704815897,7.79963077096185));
#21343=CARTESIAN_POINT('Origin',(2.36305161962877,0.,0.));
#21344=CARTESIAN_POINT('',(2.36305161962877,-2.28830166396292,7.97832535653345));
#21345=CARTESIAN_POINT('Ctrl Pts',(2.36305161962877,-2.83826704815897,7.79963077096185));
#21346=CARTESIAN_POINT('Ctrl Pts',(2.3422623536685,-2.7464656808039,7.83303706974588));
#21347=CARTESIAN_POINT('Ctrl Pts',(2.33256137669178,-2.65313425633026,7.86508088454567));
#21348=CARTESIAN_POINT('Ctrl Pts',(2.33256137669178,-2.47654785029387,7.92245728595388));
#21349=CARTESIAN_POINT('Ctrl Pts',(2.3422623536685,-2.38220626001896,7.95139213009729));
#21350=CARTESIAN_POINT('Ctrl Pts',(2.36305161962877,-2.28830166396292,7.97832535653345));
#21351=CARTESIAN_POINT('',(2.36305161962877,2.28830166396292,7.97832535653345));
#21352=CARTESIAN_POINT('Origin',(2.36305161962877,0.,0.));
#21353=CARTESIAN_POINT('',(2.36305161962877,2.83826704815898,7.79963077096185));
#21354=CARTESIAN_POINT('Ctrl Pts',(2.36305161962877,2.28830166396292,7.97832535653344));
#21355=CARTESIAN_POINT('Ctrl Pts',(2.3422623536685,2.38220626001896,7.95139213009729));
#21356=CARTESIAN_POINT('Ctrl Pts',(2.33256137669178,2.47654785029387,7.92245728595388));
#21357=CARTESIAN_POINT('Ctrl Pts',(2.33256137669178,2.65313425633026,7.86508088454567));
#21358=CARTESIAN_POINT('Ctrl Pts',(2.3422623536685,2.7464656808039,7.83303706974588));
#21359=CARTESIAN_POINT('Ctrl Pts',(2.36305161962877,2.83826704815897,7.79963077096185));
#21360=CARTESIAN_POINT('',(2.36305161962877,6.54081691696392,5.10957082921439));
#21361=CARTESIAN_POINT('Origin',(2.36305161962877,0.,0.));
#21362=CARTESIAN_POINT('',(2.36305161962877,6.88071421703298,4.64174233058237));
#21363=CARTESIAN_POINT('Ctrl Pts',(2.36305161962877,6.54081691696392,5.10957082921439));
#21364=CARTESIAN_POINT('Ctrl Pts',(2.3422623536685,6.60095637772735,5.03258565462997));
#21365=CARTESIAN_POINT('Ctrl Pts',(2.33256137669178,6.66027285287123,4.95372427854694));
#21366=CARTESIAN_POINT('Ctrl Pts',(2.33256137669178,6.7694092537529,4.80351090950811));
#21367=CARTESIAN_POINT('Ctrl Pts',(2.3422623536685,6.82608108049479,4.72272808388942));
#21368=CARTESIAN_POINT('Ctrl Pts',(2.36305161962877,6.88071421703298,4.64174233058237));
#21369=CARTESIAN_POINT('',(2.36305161962877,8.294962421875,0.289133913060419));
#21370=CARTESIAN_POINT('Origin',(2.36305161962877,0.,0.));
#21371=CARTESIAN_POINT('',(2.36305161962877,8.294962421875,-0.289133913060419));
#21372=CARTESIAN_POINT('Ctrl Pts',(2.36305161962877,8.294962421875,0.289133913060419));
#21373=CARTESIAN_POINT('Ctrl Pts',(2.3422623536685,8.29836551739928,0.191502510389135));
#21374=CARTESIAN_POINT('Ctrl Pts',(2.33256137669178,8.3,0.0928369676306301));
#21375=CARTESIAN_POINT('Ctrl Pts',(2.33256137669178,8.3,-0.09283696763063));
#21376=CARTESIAN_POINT('Ctrl Pts',(2.3422623536685,8.29836551739928,-0.191502510389135));
#21377=CARTESIAN_POINT('Ctrl Pts',(2.36305161962877,8.294962421875,-0.289133913060419));
#21378=CARTESIAN_POINT('Origin',(2.36305161962877,0.,0.));
#21379=CARTESIAN_POINT('Origin',(4.,0.,0.));
#21380=CARTESIAN_POINT('',(5.63694838037123,2.83826704815896,-7.79963077096186));
#21381=CARTESIAN_POINT('Origin',(5.63694838037123,0.,0.));
#21382=CARTESIAN_POINT('Ctrl Pts',(5.63694838037123,2.83826704815898,-7.79963077096185));
#21383=CARTESIAN_POINT('Ctrl Pts',(5.43435502838932,2.77475170678766,-7.61514961115077));
#21384=CARTESIAN_POINT('Ctrl Pts',(5.1585814386757,2.71625203654638,-7.44544836653197));
#21385=CARTESIAN_POINT('Ctrl Pts',(4.63401515068219,2.64540317647514,-7.24001881570869));
#21386=CARTESIAN_POINT('Ctrl Pts',(4.29124189438349,2.6231528858578,-7.17556053123489));
#21387=CARTESIAN_POINT('Ctrl Pts',(3.70875810561651,2.6231528858578,-7.17556053123489));
#21388=CARTESIAN_POINT('Ctrl Pts',(3.36598484931781,2.64540317647514,-7.24001881570869));
#21389=CARTESIAN_POINT('Ctrl Pts',(2.8414185613243,2.71625203654638,-7.44544836653197));
#21390=CARTESIAN_POINT('Ctrl Pts',(2.56564497161068,2.77475170678765,-7.61514961115078));
#21391=CARTESIAN_POINT('Ctrl Pts',(2.36305161962877,2.83826704815898,-7.79963077096185));
#21392=CARTESIAN_POINT('Origin',(4.,3.09016994374947,-9.51056516295154));
#21393=CARTESIAN_POINT('',(4.,5.35487327317731,-8.77471844509619));
#21394=CARTESIAN_POINT('',(4.,0.825466614321638,-10.2464118808069));
#21395=CARTESIAN_POINT('Origin',(4.,3.09016994374947,-9.51056516295154));
#21396=CARTESIAN_POINT('',(2.36305161962877,3.28744573566193,-11.2286553306742));
#21397=CARTESIAN_POINT('Ctrl Pts',(2.36305161962876,3.28744573566193,-11.2286553306742));
#21398=CARTESIAN_POINT('Ctrl Pts',(2.34215062955512,3.39935280476416,-11.1958919760002));
#21399=CARTESIAN_POINT('Ctrl Pts',(2.33256137669178,3.51096249710822,-11.1613271555422));
#21400=CARTESIAN_POINT('Ctrl Pts',(2.33256137669178,3.72003517126555,-11.0933953257644));
#21401=CARTESIAN_POINT('Ctrl Pts',(2.34215062955513,3.83064600082223,-11.0557563217497));
#21402=CARTESIAN_POINT('Ctrl Pts',(2.36305161962877,3.94043853820961,-11.0164851076281));
#21403=CARTESIAN_POINT('Ctrl Pts',(5.63694838037123,3.28744573566191,-11.2286553306742));
#21404=CARTESIAN_POINT('Ctrl Pts',(5.43435664662035,3.34500560751313,-11.4150699014315));
#21405=CARTESIAN_POINT('Ctrl Pts',(5.15858882449494,3.3979980701903,-11.586556855709));
#21406=CARTESIAN_POINT('Ctrl Pts',(4.63402456511048,3.46216697347001,-11.7941603096066));
#21407=CARTESIAN_POINT('Ctrl Pts',(4.2912458937239,3.4823124798495,-11.8593043553441));
#21408=CARTESIAN_POINT('Ctrl Pts',(4.,3.4823124798495,-11.8593043553441));
#21409=CARTESIAN_POINT('Ctrl Pts',(3.7087541062761,3.4823124798495,-11.8593043553441));
#21410=CARTESIAN_POINT('Ctrl Pts',(3.36597543488952,3.46216697347001,-11.7941603096066));
#21411=CARTESIAN_POINT('Ctrl Pts',(2.84141117550506,3.3979980701903,-11.586556855709));
#21412=CARTESIAN_POINT('Ctrl Pts',(2.56564335337965,3.34500560751313,-11.4150699014315));
#21413=CARTESIAN_POINT('Ctrl Pts',(2.36305161962877,3.28744573566191,-11.2286553306742));
#21414=CARTESIAN_POINT('',(5.63694838037123,2.28830166396294,-7.97832535653344));
#21415=CARTESIAN_POINT('Ctrl Pts',(5.63694838037124,2.28830166396294,-7.97832535653344));
#21416=CARTESIAN_POINT('Ctrl Pts',(5.6577376463315,2.38220626001897,-7.95139213009729));
#21417=CARTESIAN_POINT('Ctrl Pts',(5.66743862330822,2.47654785029387,-7.92245728595388));
#21418=CARTESIAN_POINT('Ctrl Pts',(5.66743862330822,2.65313425633025,-7.86508088454568));
#21419=CARTESIAN_POINT('Ctrl Pts',(5.6577376463315,2.74646568080388,-7.83303706974588));
#21420=CARTESIAN_POINT('Ctrl Pts',(5.63694838037124,2.83826704815896,-7.79963077096186));
#21421=CARTESIAN_POINT('Ctrl Pts',(2.36305161962877,2.28830166396291,-7.97832535653345));
#21422=CARTESIAN_POINT('Ctrl Pts',(2.56564497161068,2.23125134947308,-7.7917435821519));
#21423=CARTESIAN_POINT('Ctrl Pts',(2.8414185613243,2.17883068798099,-7.62006714785691));
#21424=CARTESIAN_POINT('Ctrl Pts',(3.36598484931781,2.11540015945172,-7.41222723500246));
#21425=CARTESIAN_POINT('Ctrl Pts',(3.70875810561651,2.09551339368916,-7.34700099475081));
#21426=CARTESIAN_POINT('Ctrl Pts',(4.29124189438349,2.09551339368916,-7.34700099475081));
#21427=CARTESIAN_POINT('Ctrl Pts',(4.63401515068219,2.11540015945172,-7.41222723500246));
#21428=CARTESIAN_POINT('Ctrl Pts',(5.1585814386757,2.17883068798099,-7.62006714785691));
#21429=CARTESIAN_POINT('Ctrl Pts',(5.43435502838932,2.23125134947308,-7.7917435821519));
#21430=CARTESIAN_POINT('Ctrl Pts',(5.63694838037123,2.28830166396291,-7.97832535653345));
#21431=CARTESIAN_POINT('Origin',(4.,0.,0.));
#21432=CARTESIAN_POINT('',(2.36305161962877,-3.28744573566193,-11.2286553306742));
#21433=CARTESIAN_POINT('Origin',(2.36305161962877,0.,0.));
#21434=CARTESIAN_POINT('Ctrl Pts',(2.36305161962877,-3.28744573566191,-11.2286553306742));
#21435=CARTESIAN_POINT('Ctrl Pts',(2.56564335337965,-3.34500560751313,-11.4150699014315));
#21436=CARTESIAN_POINT('Ctrl Pts',(2.84141117550506,-3.39799807019031,-11.586556855709));
#21437=CARTESIAN_POINT('Ctrl Pts',(3.36597543488952,-3.46216697347002,-11.7941603096066));
#21438=CARTESIAN_POINT('Ctrl Pts',(3.7087541062761,-3.48231247984951,-11.8593043553441));
#21439=CARTESIAN_POINT('Ctrl Pts',(4.,-3.48231247984951,-11.8593043553441));
#21440=CARTESIAN_POINT('Ctrl Pts',(4.2912458937239,-3.48231247984951,-11.8593043553441));
#21441=CARTESIAN_POINT('Ctrl Pts',(4.63402456511049,-3.46216697347002,-11.7941603096066));
#21442=CARTESIAN_POINT('Ctrl Pts',(5.15858882449494,-3.39799807019031,-11.586556855709));
#21443=CARTESIAN_POINT('Ctrl Pts',(5.43435664662035,-3.34500560751314,-11.4150699014315));
#21444=CARTESIAN_POINT('Ctrl Pts',(5.63694838037123,-3.28744573566191,-11.2286553306742));
#21445=CARTESIAN_POINT('Origin',(4.,0.,0.));
#21446=CARTESIAN_POINT('',(5.63694838037123,-2.28830166396294,-7.97832535653344));
#21447=CARTESIAN_POINT('Origin',(5.63694838037123,0.,0.));
#21448=CARTESIAN_POINT('Ctrl Pts',(5.63694838037123,-2.28830166396291,-7.97832535653345));
#21449=CARTESIAN_POINT('Ctrl Pts',(5.43435502838932,-2.23125134947308,-7.7917435821519));
#21450=CARTESIAN_POINT('Ctrl Pts',(5.1585814386757,-2.17883068798099,-7.62006714785691));
#21451=CARTESIAN_POINT('Ctrl Pts',(4.6340151506822,-2.11540015945172,-7.41222723500246));
#21452=CARTESIAN_POINT('Ctrl Pts',(4.29124189438349,-2.09551339368916,-7.34700099475081));
#21453=CARTESIAN_POINT('Ctrl Pts',(3.70875810561651,-2.09551339368916,-7.34700099475081));
#21454=CARTESIAN_POINT('Ctrl Pts',(3.36598484931781,-2.11540015945172,-7.41222723500246));
#21455=CARTESIAN_POINT('Ctrl Pts',(2.8414185613243,-2.17883068798099,-7.62006714785691));
#21456=CARTESIAN_POINT('Ctrl Pts',(2.56564497161068,-2.23125134947308,-7.7917435821519));
#21457=CARTESIAN_POINT('Ctrl Pts',(2.36305161962877,-2.28830166396292,-7.97832535653345));
#21458=CARTESIAN_POINT('Origin',(4.,-3.09016994374948,-9.51056516295153));
#21459=CARTESIAN_POINT('',(4.,-0.825466614321642,-10.2464118808069));
#21460=CARTESIAN_POINT('',(4.,-5.35487327317731,-8.77471844509619));
#21461=CARTESIAN_POINT('Origin',(4.,-3.09016994374948,-9.51056516295153));
#21462=CARTESIAN_POINT('',(2.36305161962877,-3.94043853820961,-11.0164851076281));
#21463=CARTESIAN_POINT('Ctrl Pts',(2.36305161962877,-3.94043853820961,-11.0164851076281));
#21464=CARTESIAN_POINT('Ctrl Pts',(2.34215062955513,-3.83064600082223,-11.0557563217497));
#21465=CARTESIAN_POINT('Ctrl Pts',(2.33256137669178,-3.72003517126555,-11.0933953257644));
#21466=CARTESIAN_POINT('Ctrl Pts',(2.33256137669178,-3.51096249710823,-11.1613271555422));
#21467=CARTESIAN_POINT('Ctrl Pts',(2.34215062955513,-3.39935280476416,-11.1958919760002));
#21468=CARTESIAN_POINT('Ctrl Pts',(2.36305161962877,-3.28744573566193,-11.2286553306742));
#21469=CARTESIAN_POINT('Ctrl Pts',(5.63694838037123,-3.94043853820963,-11.0164851076281));
#21470=CARTESIAN_POINT('Ctrl Pts',(5.43435664662035,-4.00344335919149,-11.2011305071679));
#21471=CARTESIAN_POINT('Ctrl Pts',(5.15858882449494,-4.06136905899675,-11.3710145555363));
#21472=CARTESIAN_POINT('Ctrl Pts',(4.63402456511049,-4.13148157425907,-11.576686812834));
#21473=CARTESIAN_POINT('Ctrl Pts',(4.2912458937239,-4.15347422659696,-11.6412306844678));
#21474=CARTESIAN_POINT('Ctrl Pts',(4.,-4.15347422659696,-11.6412306844678));
#21475=CARTESIAN_POINT('Ctrl Pts',(3.7087541062761,-4.15347422659696,-11.6412306844678));
#21476=CARTESIAN_POINT('Ctrl Pts',(3.36597543488952,-4.13148157425907,-11.576686812834));
#21477=CARTESIAN_POINT('Ctrl Pts',(2.84141117550506,-4.06136905899675,-11.3710145555363));
#21478=CARTESIAN_POINT('Ctrl Pts',(2.56564335337965,-4.00344335919149,-11.2011305071679));
#21479=CARTESIAN_POINT('Ctrl Pts',(2.36305161962877,-3.94043853820963,-11.0164851076281));
#21480=CARTESIAN_POINT('',(5.63694838037123,-2.83826704815896,-7.79963077096186));
#21481=CARTESIAN_POINT('Ctrl Pts',(5.63694838037124,-2.83826704815896,-7.79963077096186));
#21482=CARTESIAN_POINT('Ctrl Pts',(5.6577376463315,-2.74646568080389,-7.83303706974588));
#21483=CARTESIAN_POINT('Ctrl Pts',(5.66743862330822,-2.65313425633025,-7.86508088454567));
#21484=CARTESIAN_POINT('Ctrl Pts',(5.66743862330822,-2.47654785029388,-7.92245728595387));
#21485=CARTESIAN_POINT('Ctrl Pts',(5.6577376463315,-2.38220626001897,-7.95139213009729));
#21486=CARTESIAN_POINT('Ctrl Pts',(5.63694838037124,-2.28830166396294,-7.97832535653344));
#21487=CARTESIAN_POINT('Ctrl Pts',(2.36305161962877,-2.83826704815898,-7.79963077096185));
#21488=CARTESIAN_POINT('Ctrl Pts',(2.56564497161068,-2.77475170678766,-7.61514961115077));
#21489=CARTESIAN_POINT('Ctrl Pts',(2.8414185613243,-2.71625203654638,-7.44544836653197));
#21490=CARTESIAN_POINT('Ctrl Pts',(3.36598484931781,-2.64540317647514,-7.24001881570868));
#21491=CARTESIAN_POINT('Ctrl Pts',(3.70875810561651,-2.6231528858578,-7.17556053123489));
#21492=CARTESIAN_POINT('Ctrl Pts',(4.29124189438349,-2.6231528858578,-7.17556053123489));
#21493=CARTESIAN_POINT('Ctrl Pts',(4.63401515068219,-2.64540317647514,-7.24001881570868));
#21494=CARTESIAN_POINT('Ctrl Pts',(5.1585814386757,-2.71625203654638,-7.44544836653197));
#21495=CARTESIAN_POINT('Ctrl Pts',(5.43435502838932,-2.77475170678766,-7.61514961115077));
#21496=CARTESIAN_POINT('Ctrl Pts',(5.63694838037123,-2.83826704815898,-7.79963077096185));
#21497=CARTESIAN_POINT('Origin',(4.,0.,0.));
#21498=CARTESIAN_POINT('',(2.36305161962877,-9.25963747468151,-7.15186086536041));
#21499=CARTESIAN_POINT('Origin',(2.36305161962877,0.,0.));
#21500=CARTESIAN_POINT('Ctrl Pts',(2.36305161962877,-9.25963747468149,-7.15186086536043));
#21501=CARTESIAN_POINT('Ctrl Pts',(2.56564335337965,-9.41577612470672,-7.26884057730417));
#21502=CARTESIAN_POINT('Ctrl Pts',(2.84141117550506,-9.55944543027122,-7.37642824958397));
#21503=CARTESIAN_POINT('Ctrl Pts',(3.36597543488952,-9.73338541206091,-7.5066654368745));
#21504=CARTESIAN_POINT('Ctrl Pts',(3.7087541062761,-9.7879741784414,-7.54752684540867));
#21505=CARTESIAN_POINT('Ctrl Pts',(4.,-9.7879741784414,-7.54752684540867));
#21506=CARTESIAN_POINT('Ctrl Pts',(4.2912458937239,-9.7879741784414,-7.54752684540867));
#21507=CARTESIAN_POINT('Ctrl Pts',(4.63402456511048,-9.73338541206091,-7.5066654368745));
#21508=CARTESIAN_POINT('Ctrl Pts',(5.15858882449494,-9.55944543027122,-7.37642824958397));
#21509=CARTESIAN_POINT('Ctrl Pts',(5.43435664662035,-9.41577612470672,-7.26884057730417));
#21510=CARTESIAN_POINT('Ctrl Pts',(5.63694838037123,-9.2596374746815,-7.15186086536043));
#21511=CARTESIAN_POINT('Origin',(4.,0.,0.));
#21512=CARTESIAN_POINT('',(5.63694838037123,-6.54081691696393,-5.10957082921437));
#21513=CARTESIAN_POINT('Origin',(5.63694838037123,0.,0.));
#21514=CARTESIAN_POINT('Ctrl Pts',(5.63694838037123,-6.54081691696392,-5.10957082921439));
#21515=CARTESIAN_POINT('Ctrl Pts',(5.43435502838932,-6.38499222767917,-4.99215633639485));
#21516=CARTESIAN_POINT('Ctrl Pts',(5.1585814386757,-6.24167414543093,-4.884079275257));
#21517=CARTESIAN_POINT('Ctrl Pts',(4.63401515068219,-6.06819253427497,-4.75321678286296));
#21518=CARTESIAN_POINT('Ctrl Pts',(4.29124189438349,-6.01376478072751,-4.7121367936512));
#21519=CARTESIAN_POINT('Ctrl Pts',(3.70875810561651,-6.01376478072751,-4.7121367936512));
#21520=CARTESIAN_POINT('Ctrl Pts',(3.36598484931781,-6.06819253427498,-4.75321678286295));
#21521=CARTESIAN_POINT('Ctrl Pts',(2.8414185613243,-6.24167414543094,-4.88407927525699));
#21522=CARTESIAN_POINT('Ctrl Pts',(2.56564497161068,-6.38499222767918,-4.99215633639486));
#21523=CARTESIAN_POINT('Ctrl Pts',(2.36305161962877,-6.54081691696392,-5.10957082921439));
#21524=CARTESIAN_POINT('Origin',(4.,-8.09016994374948,-5.87785252292473));
#21525=CARTESIAN_POINT('',(4.,-6.69050631172802,-7.80432424078007));
#21526=CARTESIAN_POINT('',(4.,-9.48983357577093,-3.95138080506939));
#21527=CARTESIAN_POINT('Origin',(4.,-8.09016994374948,-5.87785252292473));
#21528=CARTESIAN_POINT('',(2.36305161962877,-9.66320922106503,-6.59639201002516));
#21529=CARTESIAN_POINT('Ctrl Pts',(2.36305161962876,-9.66320922106503,-6.59639201002516));
#21530=CARTESIAN_POINT('Ctrl Pts',(2.34215062955512,-9.59746823296338,-6.69269752392734));
#21531=CARTESIAN_POINT('Ctrl Pts',(2.33256137669178,-9.53010584356091,-6.78816353218381));
#21532=CARTESIAN_POINT('Ctrl Pts',(2.33256137669178,-9.40089182481285,-6.96601137146006));
#21533=CARTESIAN_POINT('Ctrl Pts',(2.34215062955512,-9.33091437868292,-7.05957742979088));
#21534=CARTESIAN_POINT('Ctrl Pts',(2.36305161962876,-9.25963747468151,-7.15186086536041));
#21535=CARTESIAN_POINT('Ctrl Pts',(5.63694838037123,-9.66320922106504,-6.59639201002514));
#21536=CARTESIAN_POINT('Ctrl Pts',(5.43435664662035,-9.82271303472002,-6.70873997158946));
#21537=CARTESIAN_POINT('Ctrl Pts',(5.15858882449494,-9.96943124850423,-6.81213118171847));
#21538=CARTESIAN_POINT('Ctrl Pts',(4.63402456511048,-10.1470445845151,-6.93731243067146));
#21539=CARTESIAN_POINT('Ctrl Pts',(4.2912458937239,-10.2027749498801,-6.97660256300298));
#21540=CARTESIAN_POINT('Ctrl Pts',(4.,-10.2027749498801,-6.97660256300298));
#21541=CARTESIAN_POINT('Ctrl Pts',(3.7087541062761,-10.2027749498801,-6.97660256300298));
#21542=CARTESIAN_POINT('Ctrl Pts',(3.36597543488952,-10.1470445845151,-6.93731243067146));
#21543=CARTESIAN_POINT('Ctrl Pts',(2.84141117550507,-9.96943124850423,-6.81213118171847));
#21544=CARTESIAN_POINT('Ctrl Pts',(2.56564335337965,-9.82271303472002,-6.70873997158947));
#21545=CARTESIAN_POINT('Ctrl Pts',(2.36305161962877,-9.66320922106504,-6.59639201002514));
#21546=CARTESIAN_POINT('',(5.63694838037123,-6.88071421703297,-4.64174233058239));
#21547=CARTESIAN_POINT('Ctrl Pts',(5.63694838037124,-6.88071421703297,-4.64174233058239));
#21548=CARTESIAN_POINT('Ctrl Pts',(5.6577376463315,-6.82608108049478,-4.72272808388943));
#21549=CARTESIAN_POINT('Ctrl Pts',(5.66743862330822,-6.7694092537529,-4.80351090950812));
#21550=CARTESIAN_POINT('Ctrl Pts',(5.66743862330822,-6.66027285287123,-4.95372427854694));
#21551=CARTESIAN_POINT('Ctrl Pts',(5.6577376463315,-6.60095637772736,-5.03258565462996));
#21552=CARTESIAN_POINT('Ctrl Pts',(5.63694838037124,-6.54081691696393,-5.10957082921437));
#21553=CARTESIAN_POINT('Ctrl Pts',(2.36305161962877,-6.88071421703298,-4.64174233058237));
#21554=CARTESIAN_POINT('Ctrl Pts',(2.56564497161068,-6.72089392139729,-4.5298273181056));
#21555=CARTESIAN_POINT('Ctrl Pts',(2.8414185613243,-6.57381880512416,-4.4269213706742));
#21556=CARTESIAN_POINT('Ctrl Pts',(3.36598484931781,-6.39575241293544,-4.30236928800296));
#21557=CARTESIAN_POINT('Ctrl Pts',(3.70875810561651,-6.33986392069446,-4.26329983311949));
#21558=CARTESIAN_POINT('Ctrl Pts',(4.29124189438349,-6.33986392069446,-4.26329983311949));
#21559=CARTESIAN_POINT('Ctrl Pts',(4.63401515068219,-6.39575241293545,-4.30236928800294));
#21560=CARTESIAN_POINT('Ctrl Pts',(5.1585814386757,-6.57381880512417,-4.42692137067418));
#21561=CARTESIAN_POINT('Ctrl Pts',(5.43435502838932,-6.72089392139729,-4.5298273181056));
#21562=CARTESIAN_POINT('Ctrl Pts',(5.63694838037123,-6.88071421703298,-4.64174233058237));
#21563=CARTESIAN_POINT('Origin',(4.,0.,0.));
#21564=CARTESIAN_POINT('',(2.36305161962877,-11.694962421875,-0.343298632289181));
#21565=CARTESIAN_POINT('Origin',(2.36305161962877,0.,0.));
#21566=CARTESIAN_POINT('Ctrl Pts',(2.36305161962877,-11.694962421875,-0.3432986322892));
#21567=CARTESIAN_POINT('Ctrl Pts',(2.56564335337965,-11.8900401927221,-0.34616121145108));
#21568=CARTESIAN_POINT('Ctrl Pts',(2.84141117550506,-12.0695095495884,-0.348754767692782));
#21569=CARTESIAN_POINT('Ctrl Pts',(3.36597543488952,-12.2867814488469,-0.351879509430404));
#21570=CARTESIAN_POINT('Ctrl Pts',(3.7087541062761,-12.354962421875,-0.352850611529358));
#21571=CARTESIAN_POINT('Ctrl Pts',(4.,-12.354962421875,-0.352850611529358));
#21572=CARTESIAN_POINT('Ctrl Pts',(4.2912458937239,-12.354962421875,-0.352850611529358));
#21573=CARTESIAN_POINT('Ctrl Pts',(4.63402456511048,-12.2867814488469,-0.351879509430404));
#21574=CARTESIAN_POINT('Ctrl Pts',(5.15858882449494,-12.0695095495884,-0.348754767692782));
#21575=CARTESIAN_POINT('Ctrl Pts',(5.43435664662035,-11.8900401927221,-0.34616121145108));
#21576=CARTESIAN_POINT('Ctrl Pts',(5.63694838037123,-11.694962421875,-0.343298632289199));
#21577=CARTESIAN_POINT('Origin',(4.,0.,0.));
#21578=CARTESIAN_POINT('',(5.63694838037123,-8.294962421875,-0.289133913060398));
#21579=CARTESIAN_POINT('Origin',(5.63694838037123,0.,0.));
#21580=CARTESIAN_POINT('Ctrl Pts',(5.63694838037123,-8.294962421875,-0.28913391306042));
#21581=CARTESIAN_POINT('Ctrl Pts',(5.43435502838932,-8.09988309281573,-0.285735047288132));
#21582=CARTESIAN_POINT('Ctrl Pts',(5.1585814386757,-7.92041022602772,-0.282539123257846));
#21583=CARTESIAN_POINT('Ctrl Pts',(4.63401515068219,-7.70314161128355,-0.278639075566217));
#21584=CARTESIAN_POINT('Ctrl Pts',(4.29124189438349,-7.634962421875,-0.277396497015791));
#21585=CARTESIAN_POINT('Ctrl Pts',(3.70875810561651,-7.634962421875,-0.277396497015791));
#21586=CARTESIAN_POINT('Ctrl Pts',(3.36598484931781,-7.70314161128355,-0.278639075566217));
#21587=CARTESIAN_POINT('Ctrl Pts',(2.8414185613243,-7.92041022602773,-0.282539123257846));
#21588=CARTESIAN_POINT('Ctrl Pts',(2.56564497161068,-8.09988309281573,-0.285735047288137));
#21589=CARTESIAN_POINT('Ctrl Pts',(2.36305161962877,-8.294962421875,-0.289133913060424));
#21590=CARTESIAN_POINT('Origin',(4.,-10.,1.22464679914735E-15));
#21591=CARTESIAN_POINT('',(4.,-10.,-2.38125));
#21592=CARTESIAN_POINT('',(4.,-10.,2.38125));
#21593=CARTESIAN_POINT('Origin',(4.,-10.,1.22464679914735E-15));
#21594=CARTESIAN_POINT('',(2.36305161962877,-11.694962421875,0.343298632289184));
#21595=CARTESIAN_POINT('',(2.33256137669178,-11.7,-5.72234566300149E-17));
#21596=CARTESIAN_POINT('Ctrl Pts',(2.36305161962876,-11.694962421875,0.343298632289185));
#21597=CARTESIAN_POINT('Ctrl Pts',(2.34215062955512,-11.6983838060599,0.226744251613028));
#21598=CARTESIAN_POINT('Ctrl Pts',(2.33256137669178,-11.7,0.109916009498454));
#21599=CARTESIAN_POINT('Ctrl Pts',(2.33256137669178,-11.7,1.28369537222284E-15));
#21600=CARTESIAN_POINT('Ctrl Pts',(5.63694838037123,-11.694962421875,0.343298632289202));
#21601=CARTESIAN_POINT('Ctrl Pts',(5.43435664662035,-11.8900401927221,0.346161211451083));
#21602=CARTESIAN_POINT('Ctrl Pts',(5.15858882449494,-12.0695095495884,0.348754767692785));
#21603=CARTESIAN_POINT('Ctrl Pts',(4.63402456511048,-12.2867814488469,0.351879509430407));
#21604=CARTESIAN_POINT('Ctrl Pts',(4.2912458937239,-12.354962421875,0.352850611529361));
#21605=CARTESIAN_POINT('Ctrl Pts',(4.,-12.354962421875,0.352850611529361));
#21606=CARTESIAN_POINT('Ctrl Pts',(3.7087541062761,-12.354962421875,0.352850611529361));
#21607=CARTESIAN_POINT('Ctrl Pts',(3.36597543488952,-12.2867814488469,0.351879509430407));
#21608=CARTESIAN_POINT('Ctrl Pts',(2.84141117550506,-12.0695095495884,0.348754767692785));
#21609=CARTESIAN_POINT('Ctrl Pts',(2.56564335337965,-11.8900401927221,0.346161211451082));
#21610=CARTESIAN_POINT('Ctrl Pts',(2.36305161962877,-11.694962421875,0.343298632289202));
#21611=CARTESIAN_POINT('Ctrl Pts',(2.33256137669178,-11.7,1.31838984174237E-15));
#21612=CARTESIAN_POINT('Ctrl Pts',(2.33256137669178,-11.7,-0.109916009498451));
#21613=CARTESIAN_POINT('Ctrl Pts',(2.34215062955512,-11.6983838060599,-0.226744251613025));
#21614=CARTESIAN_POINT('Ctrl Pts',(2.36305161962876,-11.694962421875,-0.343298632289182));
#21615=CARTESIAN_POINT('',(5.63694838037123,-8.294962421875,0.2891339130604));
#21616=CARTESIAN_POINT('',(5.66743862330822,-8.3,-1.0503295078889E-15));
#21617=CARTESIAN_POINT('Ctrl Pts',(5.63694838037124,-8.294962421875,0.289133913060401));
#21618=CARTESIAN_POINT('Ctrl Pts',(5.6577376463315,-8.29836551739928,0.191502510389123));
#21619=CARTESIAN_POINT('Ctrl Pts',(5.66743862330822,-8.3,0.092836967630624));
#21620=CARTESIAN_POINT('Ctrl Pts',(5.66743862330822,-8.3,-1.0842021724855E-15));
#21621=CARTESIAN_POINT('Ctrl Pts',(2.36305161962877,-8.294962421875,0.289133913060426));
#21622=CARTESIAN_POINT('Ctrl Pts',(2.56564497161068,-8.09988309281573,0.285735047288139));
#21623=CARTESIAN_POINT('Ctrl Pts',(2.8414185613243,-7.92041022602773,0.282539123257848));
#21624=CARTESIAN_POINT('Ctrl Pts',(3.36598484931781,-7.70314161128355,0.278639075566219));
#21625=CARTESIAN_POINT('Ctrl Pts',(3.70875810561651,-7.634962421875,0.277396497015793));
#21626=CARTESIAN_POINT('Ctrl Pts',(4.29124189438349,-7.634962421875,0.277396497015793));
#21627=CARTESIAN_POINT('Ctrl Pts',(4.63401515068219,-7.70314161128355,0.278639075566219));
#21628=CARTESIAN_POINT('Ctrl Pts',(5.1585814386757,-7.92041022602772,0.282539123257848));
#21629=CARTESIAN_POINT('Ctrl Pts',(5.43435502838932,-8.09988309281573,0.285735047288134));
#21630=CARTESIAN_POINT('Ctrl Pts',(5.63694838037123,-8.294962421875,0.289133913060422));
#21631=CARTESIAN_POINT('Ctrl Pts',(5.66743862330822,-8.3,-1.0842021724855E-15));
#21632=CARTESIAN_POINT('Ctrl Pts',(5.66743862330822,-8.3,-0.0928369676306247));
#21633=CARTESIAN_POINT('Ctrl Pts',(5.6577376463315,-8.29836551739928,-0.191502510389122));
#21634=CARTESIAN_POINT('Ctrl Pts',(5.63694838037124,-8.294962421875,-0.289133913060399));
#21635=CARTESIAN_POINT('Origin',(4.,0.,0.));
#21636=CARTESIAN_POINT('',(2.36305161962877,-9.66320922106502,6.59639201002516));
#21637=CARTESIAN_POINT('Origin',(2.36305161962877,0.,0.));
#21638=CARTESIAN_POINT('Ctrl Pts',(2.36305161962877,-9.66320922106503,6.59639201002515));
#21639=CARTESIAN_POINT('Ctrl Pts',(2.56564335337965,-9.82271303472001,6.70873997158947));
#21640=CARTESIAN_POINT('Ctrl Pts',(2.84141117550506,-9.96943124850423,6.81213118171848));
#21641=CARTESIAN_POINT('Ctrl Pts',(3.36597543488952,-10.1470445845151,6.93731243067146));
#21642=CARTESIAN_POINT('Ctrl Pts',(3.7087541062761,-10.2027749498801,6.97660256300298));
#21643=CARTESIAN_POINT('Ctrl Pts',(4.,-10.2027749498801,6.97660256300298));
#21644=CARTESIAN_POINT('Ctrl Pts',(4.2912458937239,-10.2027749498801,6.97660256300298));
#21645=CARTESIAN_POINT('Ctrl Pts',(4.63402456511048,-10.1470445845151,6.93731243067146));
#21646=CARTESIAN_POINT('Ctrl Pts',(5.15858882449494,-9.96943124850423,6.81213118171848));
#21647=CARTESIAN_POINT('Ctrl Pts',(5.43435664662035,-9.82271303472001,6.70873997158947));
#21648=CARTESIAN_POINT('Ctrl Pts',(5.63694838037123,-9.66320922106503,6.59639201002515));
#21649=CARTESIAN_POINT('Origin',(4.,0.,0.));
#21650=CARTESIAN_POINT('',(5.63694838037123,-6.88071421703296,4.64174233058239));
#21651=CARTESIAN_POINT('Origin',(5.63694838037123,0.,0.));
#21652=CARTESIAN_POINT('Ctrl Pts',(5.63694838037123,-6.88071421703298,4.64174233058237));
#21653=CARTESIAN_POINT('Ctrl Pts',(5.43435502838932,-6.72089392139729,4.5298273181056));
#21654=CARTESIAN_POINT('Ctrl Pts',(5.1585814386757,-6.57381880512416,4.4269213706742));
#21655=CARTESIAN_POINT('Ctrl Pts',(4.6340151506822,-6.39575241293544,4.30236928800296));
#21656=CARTESIAN_POINT('Ctrl Pts',(4.29124189438349,-6.33986392069446,4.26329983311949));
#21657=CARTESIAN_POINT('Ctrl Pts',(3.70875810561651,-6.33986392069446,4.26329983311949));
#21658=CARTESIAN_POINT('Ctrl Pts',(3.36598484931781,-6.39575241293544,4.30236928800296));
#21659=CARTESIAN_POINT('Ctrl Pts',(2.8414185613243,-6.57381880512416,4.4269213706742));
#21660=CARTESIAN_POINT('Ctrl Pts',(2.56564497161068,-6.72089392139729,4.5298273181056));
#21661=CARTESIAN_POINT('Ctrl Pts',(2.36305161962877,-6.88071421703298,4.64174233058237));
#21662=CARTESIAN_POINT('Origin',(4.,-8.09016994374947,5.87785252292473));
#21663=CARTESIAN_POINT('',(4.,-9.48983357577093,3.95138080506939));
#21664=CARTESIAN_POINT('',(4.,-6.69050631172802,7.80432424078008));
#21665=CARTESIAN_POINT('Origin',(4.,-8.09016994374947,5.87785252292473));
#21666=CARTESIAN_POINT('',(2.36305161962877,-9.25963747468151,7.15186086536042));
#21667=CARTESIAN_POINT('Ctrl Pts',(2.36305161962876,-9.25963747468151,7.15186086536042));
#21668=CARTESIAN_POINT('Ctrl Pts',(2.34215062955512,-9.33091437868292,7.05957742979088));
#21669=CARTESIAN_POINT('Ctrl Pts',(2.33256137669178,-9.40089182481285,6.96601137146006));
#21670=CARTESIAN_POINT('Ctrl Pts',(2.33256137669178,-9.53010584356091,6.78816353218381));
#21671=CARTESIAN_POINT('Ctrl Pts',(2.34215062955513,-9.59746823296338,6.69269752392735));
#21672=CARTESIAN_POINT('Ctrl Pts',(2.36305161962877,-9.66320922106503,6.59639201002516));
#21673=CARTESIAN_POINT('Ctrl Pts',(5.63694838037123,-9.2596374746815,7.15186086536043));
#21674=CARTESIAN_POINT('Ctrl Pts',(5.43435664662035,-9.41577612470673,7.26884057730416));
#21675=CARTESIAN_POINT('Ctrl Pts',(5.15858882449494,-9.55944543027121,7.37642824958397));
#21676=CARTESIAN_POINT('Ctrl Pts',(4.63402456511048,-9.73338541206091,7.5066654368745));
#21677=CARTESIAN_POINT('Ctrl Pts',(4.2912458937239,-9.7879741784414,7.54752684540867));
#21678=CARTESIAN_POINT('Ctrl Pts',(4.,-9.7879741784414,7.54752684540867));
#21679=CARTESIAN_POINT('Ctrl Pts',(3.7087541062761,-9.7879741784414,7.54752684540867));
#21680=CARTESIAN_POINT('Ctrl Pts',(3.36597543488952,-9.73338541206091,7.5066654368745));
#21681=CARTESIAN_POINT('Ctrl Pts',(2.84141117550507,-9.55944543027121,7.37642824958397));
#21682=CARTESIAN_POINT('Ctrl Pts',(2.56564335337965,-9.41577612470673,7.26884057730416));
#21683=CARTESIAN_POINT('Ctrl Pts',(2.36305161962877,-9.2596374746815,7.15186086536043));
#21684=CARTESIAN_POINT('',(5.63694838037123,-6.54081691696393,5.10957082921437));
#21685=CARTESIAN_POINT('Ctrl Pts',(5.63694838037124,-6.54081691696393,5.10957082921438));
#21686=CARTESIAN_POINT('Ctrl Pts',(5.6577376463315,-6.60095637772735,5.03258565462996));
#21687=CARTESIAN_POINT('Ctrl Pts',(5.66743862330822,-6.66027285287123,4.95372427854694));
#21688=CARTESIAN_POINT('Ctrl Pts',(5.66743862330822,-6.7694092537529,4.80351090950812));
#21689=CARTESIAN_POINT('Ctrl Pts',(5.6577376463315,-6.82608108049478,4.72272808388943));
#21690=CARTESIAN_POINT('Ctrl Pts',(5.63694838037124,-6.88071421703297,4.64174233058239));
#21691=CARTESIAN_POINT('Ctrl Pts',(2.36305161962877,-6.54081691696391,5.10957082921439));
#21692=CARTESIAN_POINT('Ctrl Pts',(2.56564497161068,-6.38499222767917,4.99215633639486));
#21693=CARTESIAN_POINT('Ctrl Pts',(2.8414185613243,-6.24167414543094,4.88407927525699));
#21694=CARTESIAN_POINT('Ctrl Pts',(3.36598484931781,-6.06819253427498,4.75321678286295));
#21695=CARTESIAN_POINT('Ctrl Pts',(3.70875810561651,-6.0137647807275,4.7121367936512));
#21696=CARTESIAN_POINT('Ctrl Pts',(4.29124189438349,-6.0137647807275,4.7121367936512));
#21697=CARTESIAN_POINT('Ctrl Pts',(4.6340151506822,-6.06819253427498,4.75321678286295));
#21698=CARTESIAN_POINT('Ctrl Pts',(5.1585814386757,-6.24167414543094,4.88407927525699));
#21699=CARTESIAN_POINT('Ctrl Pts',(5.43435502838932,-6.38499222767917,4.99215633639486));
#21700=CARTESIAN_POINT('Ctrl Pts',(5.63694838037123,-6.54081691696391,5.10957082921439));
#21701=CARTESIAN_POINT('Origin',(4.,0.,0.));
#21702=CARTESIAN_POINT('',(2.36305161962877,-3.94043853820961,11.0164851076281));
#21703=CARTESIAN_POINT('Origin',(2.36305161962877,0.,0.));
#21704=CARTESIAN_POINT('Ctrl Pts',(2.36305161962877,-3.94043853820963,11.0164851076281));
#21705=CARTESIAN_POINT('Ctrl Pts',(2.56564335337965,-4.00344335919149,11.2011305071679));
#21706=CARTESIAN_POINT('Ctrl Pts',(2.84141117550506,-4.06136905899675,11.3710145555363));
#21707=CARTESIAN_POINT('Ctrl Pts',(3.36597543488952,-4.13148157425907,11.576686812834));
#21708=CARTESIAN_POINT('Ctrl Pts',(3.7087541062761,-4.15347422659696,11.6412306844678));
#21709=CARTESIAN_POINT('Ctrl Pts',(4.,-4.15347422659696,11.6412306844678));
#21710=CARTESIAN_POINT('Ctrl Pts',(4.2912458937239,-4.15347422659696,11.6412306844678));
#21711=CARTESIAN_POINT('Ctrl Pts',(4.63402456511048,-4.13148157425907,11.576686812834));
#21712=CARTESIAN_POINT('Ctrl Pts',(5.15858882449494,-4.06136905899675,11.3710145555363));
#21713=CARTESIAN_POINT('Ctrl Pts',(5.43435664662035,-4.00344335919149,11.2011305071678));
#21714=CARTESIAN_POINT('Ctrl Pts',(5.63694838037123,-3.94043853820963,11.0164851076281));
#21715=CARTESIAN_POINT('Origin',(4.,0.,0.));
#21716=CARTESIAN_POINT('',(5.63694838037123,-2.83826704815896,7.79963077096186));
#21717=CARTESIAN_POINT('Origin',(5.63694838037123,0.,0.));
#21718=CARTESIAN_POINT('Ctrl Pts',(5.63694838037123,-2.83826704815898,7.79963077096185));
#21719=CARTESIAN_POINT('Ctrl Pts',(5.43435502838932,-2.77475170678765,7.61514961115077));
#21720=CARTESIAN_POINT('Ctrl Pts',(5.1585814386757,-2.71625203654638,7.44544836653197));
#21721=CARTESIAN_POINT('Ctrl Pts',(4.63401515068219,-2.64540317647514,7.24001881570869));
#21722=CARTESIAN_POINT('Ctrl Pts',(4.29124189438349,-2.6231528858578,7.17556053123489));
#21723=CARTESIAN_POINT('Ctrl Pts',(3.70875810561651,-2.6231528858578,7.17556053123489));
#21724=CARTESIAN_POINT('Ctrl Pts',(3.36598484931781,-2.64540317647514,7.24001881570869));
#21725=CARTESIAN_POINT('Ctrl Pts',(2.8414185613243,-2.71625203654638,7.44544836653197));
#21726=CARTESIAN_POINT('Ctrl Pts',(2.56564497161068,-2.77475170678766,7.61514961115078));
#21727=CARTESIAN_POINT('Ctrl Pts',(2.36305161962877,-2.83826704815898,7.79963077096185));
#21728=CARTESIAN_POINT('Origin',(4.,-3.09016994374947,9.51056516295154));
#21729=CARTESIAN_POINT('',(4.,-5.35487327317731,8.77471844509619));
#21730=CARTESIAN_POINT('',(4.,-0.82546661432164,10.2464118808069));
#21731=CARTESIAN_POINT('Origin',(4.,-3.09016994374947,9.51056516295154));
#21732=CARTESIAN_POINT('',(2.36305161962877,-3.28744573566193,11.2286553306742));
#21733=CARTESIAN_POINT('Ctrl Pts',(2.36305161962876,-3.28744573566193,11.2286553306742));
#21734=CARTESIAN_POINT('Ctrl Pts',(2.34215062955512,-3.39935280476416,11.1958919760002));
#21735=CARTESIAN_POINT('Ctrl Pts',(2.33256137669178,-3.51096249710822,11.1613271555422));
#21736=CARTESIAN_POINT('Ctrl Pts',(2.33256137669178,-3.72003517126555,11.0933953257644));
#21737=CARTESIAN_POINT('Ctrl Pts',(2.34215062955512,-3.83064600082223,11.0557563217497));
#21738=CARTESIAN_POINT('Ctrl Pts',(2.36305161962876,-3.94043853820961,11.0164851076281));
#21739=CARTESIAN_POINT('Ctrl Pts',(5.63694838037123,-3.28744573566191,11.2286553306742));
#21740=CARTESIAN_POINT('Ctrl Pts',(5.43435664662035,-3.34500560751313,11.4150699014315));
#21741=CARTESIAN_POINT('Ctrl Pts',(5.15858882449494,-3.3979980701903,11.586556855709));
#21742=CARTESIAN_POINT('Ctrl Pts',(4.63402456511048,-3.46216697347001,11.7941603096066));
#21743=CARTESIAN_POINT('Ctrl Pts',(4.2912458937239,-3.4823124798495,11.8593043553441));
#21744=CARTESIAN_POINT('Ctrl Pts',(4.,-3.4823124798495,11.8593043553441));
#21745=CARTESIAN_POINT('Ctrl Pts',(3.7087541062761,-3.4823124798495,11.8593043553441));
#21746=CARTESIAN_POINT('Ctrl Pts',(3.36597543488952,-3.46216697347001,11.7941603096066));
#21747=CARTESIAN_POINT('Ctrl Pts',(2.84141117550506,-3.3979980701903,11.586556855709));
#21748=CARTESIAN_POINT('Ctrl Pts',(2.56564335337965,-3.34500560751314,11.4150699014315));
#21749=CARTESIAN_POINT('Ctrl Pts',(2.36305161962877,-3.28744573566191,11.2286553306742));
#21750=CARTESIAN_POINT('',(5.63694838037123,-2.28830166396294,7.97832535653344));
#21751=CARTESIAN_POINT('Ctrl Pts',(5.63694838037124,-2.28830166396294,7.97832535653344));
#21752=CARTESIAN_POINT('Ctrl Pts',(5.6577376463315,-2.38220626001897,7.95139213009729));
#21753=CARTESIAN_POINT('Ctrl Pts',(5.66743862330822,-2.47654785029387,7.92245728595388));
#21754=CARTESIAN_POINT('Ctrl Pts',(5.66743862330822,-2.65313425633025,7.86508088454568));
#21755=CARTESIAN_POINT('Ctrl Pts',(5.6577376463315,-2.74646568080388,7.83303706974588));
#21756=CARTESIAN_POINT('Ctrl Pts',(5.63694838037124,-2.83826704815896,7.79963077096186));
#21757=CARTESIAN_POINT('Ctrl Pts',(2.36305161962877,-2.28830166396291,7.97832535653345));
#21758=CARTESIAN_POINT('Ctrl Pts',(2.56564497161068,-2.23125134947308,7.7917435821519));
#21759=CARTESIAN_POINT('Ctrl Pts',(2.8414185613243,-2.17883068798099,7.62006714785691));
#21760=CARTESIAN_POINT('Ctrl Pts',(3.36598484931781,-2.11540015945172,7.41222723500246));
#21761=CARTESIAN_POINT('Ctrl Pts',(3.70875810561651,-2.09551339368916,7.34700099475081));
#21762=CARTESIAN_POINT('Ctrl Pts',(4.29124189438349,-2.09551339368916,7.34700099475081));
#21763=CARTESIAN_POINT('Ctrl Pts',(4.63401515068219,-2.11540015945172,7.41222723500246));
#21764=CARTESIAN_POINT('Ctrl Pts',(5.1585814386757,-2.17883068798099,7.62006714785691));
#21765=CARTESIAN_POINT('Ctrl Pts',(5.43435502838932,-2.23125134947309,7.7917435821519));
#21766=CARTESIAN_POINT('Ctrl Pts',(5.63694838037123,-2.28830166396292,7.97832535653345));
#21767=CARTESIAN_POINT('Origin',(4.,0.,0.));
#21768=CARTESIAN_POINT('',(2.36305161962877,3.28744573566193,11.2286553306742));
#21769=CARTESIAN_POINT('Origin',(2.36305161962877,0.,0.));
#21770=CARTESIAN_POINT('Ctrl Pts',(2.36305161962877,3.2874457356619,11.2286553306742));
#21771=CARTESIAN_POINT('Ctrl Pts',(2.56564335337965,3.34500560751313,11.4150699014315));
#21772=CARTESIAN_POINT('Ctrl Pts',(2.84141117550507,3.39799807019037,11.586556855709));
#21773=CARTESIAN_POINT('Ctrl Pts',(3.36597543488952,3.46216697347008,11.7941603096066));
#21774=CARTESIAN_POINT('Ctrl Pts',(3.7087541062761,3.48231247984951,11.8593043553441));
#21775=CARTESIAN_POINT('Ctrl Pts',(4.,3.48231247984951,11.8593043553441));
#21776=CARTESIAN_POINT('Ctrl Pts',(4.2912458937239,3.48231247984951,11.8593043553441));
#21777=CARTESIAN_POINT('Ctrl Pts',(4.63402456511048,3.46216697347008,11.7941603096066));
#21778=CARTESIAN_POINT('Ctrl Pts',(5.15858882449494,3.39799807019037,11.586556855709));
#21779=CARTESIAN_POINT('Ctrl Pts',(5.43435664662035,3.34500560751313,11.4150699014315));
#21780=CARTESIAN_POINT('Ctrl Pts',(5.63694838037123,3.2874457356619,11.2286553306742));
#21781=CARTESIAN_POINT('Origin',(4.,0.,0.));
#21782=CARTESIAN_POINT('',(5.63694838037123,2.28830166396294,7.97832535653344));
#21783=CARTESIAN_POINT('Origin',(5.63694838037123,0.,0.));
#21784=CARTESIAN_POINT('Ctrl Pts',(5.63694838037123,2.28830166396292,7.97832535653345));
#21785=CARTESIAN_POINT('Ctrl Pts',(5.43435502838932,2.23125134947309,7.7917435821519));
#21786=CARTESIAN_POINT('Ctrl Pts',(5.1585814386757,2.17883068798099,7.62006714785691));
#21787=CARTESIAN_POINT('Ctrl Pts',(4.6340151506822,2.11540015945172,7.41222723500246));
#21788=CARTESIAN_POINT('Ctrl Pts',(4.29124189438349,2.09551339368916,7.34700099475081));
#21789=CARTESIAN_POINT('Ctrl Pts',(3.70875810561651,2.09551339368916,7.34700099475081));
#21790=CARTESIAN_POINT('Ctrl Pts',(3.36598484931781,2.11540015945172,7.41222723500246));
#21791=CARTESIAN_POINT('Ctrl Pts',(2.8414185613243,2.17883068798099,7.62006714785691));
#21792=CARTESIAN_POINT('Ctrl Pts',(2.56564497161068,2.23125134947309,7.7917435821519));
#21793=CARTESIAN_POINT('Ctrl Pts',(2.36305161962877,2.28830166396292,7.97832535653345));
#21794=CARTESIAN_POINT('Origin',(4.,3.09016994374947,9.51056516295154));
#21795=CARTESIAN_POINT('',(4.,0.825466614321642,10.2464118808069));
#21796=CARTESIAN_POINT('',(4.,5.35487327317731,8.77471844509619));
#21797=CARTESIAN_POINT('Origin',(4.,3.09016994374947,9.51056516295154));
#21798=CARTESIAN_POINT('',(2.36305161962877,3.94043853820961,11.0164851076281));
#21799=CARTESIAN_POINT('Ctrl Pts',(2.36305161962876,3.94043853820961,11.0164851076281));
#21800=CARTESIAN_POINT('Ctrl Pts',(2.34215062955512,3.83064600082223,11.0557563217497));
#21801=CARTESIAN_POINT('Ctrl Pts',(2.33256137669178,3.72003517126555,11.0933953257644));
#21802=CARTESIAN_POINT('Ctrl Pts',(2.33256137669178,3.51096249710822,11.1613271555422));
#21803=CARTESIAN_POINT('Ctrl Pts',(2.34215062955512,3.39935280476416,11.1958919760002));
#21804=CARTESIAN_POINT('Ctrl Pts',(2.36305161962876,3.28744573566193,11.2286553306742));
#21805=CARTESIAN_POINT('Ctrl Pts',(5.63694838037123,3.94043853820963,11.0164851076281));
#21806=CARTESIAN_POINT('Ctrl Pts',(5.43435664662035,4.00344335919149,11.2011305071679));
#21807=CARTESIAN_POINT('Ctrl Pts',(5.15858882449494,4.06136905899669,11.3710145555363));
#21808=CARTESIAN_POINT('Ctrl Pts',(4.63402456511048,4.13148157425901,11.576686812834));
#21809=CARTESIAN_POINT('Ctrl Pts',(4.2912458937239,4.15347422659696,11.6412306844678));
#21810=CARTESIAN_POINT('Ctrl Pts',(4.,4.15347422659696,11.6412306844678));
#21811=CARTESIAN_POINT('Ctrl Pts',(3.7087541062761,4.15347422659696,11.6412306844678));
#21812=CARTESIAN_POINT('Ctrl Pts',(3.36597543488952,4.13148157425901,11.576686812834));
#21813=CARTESIAN_POINT('Ctrl Pts',(2.84141117550507,4.06136905899669,11.3710145555363));
#21814=CARTESIAN_POINT('Ctrl Pts',(2.56564335337965,4.00344335919149,11.2011305071678));
#21815=CARTESIAN_POINT('Ctrl Pts',(2.36305161962877,3.94043853820963,11.0164851076281));
#21816=CARTESIAN_POINT('',(5.63694838037123,2.83826704815896,7.79963077096186));
#21817=CARTESIAN_POINT('Ctrl Pts',(5.63694838037124,2.83826704815896,7.79963077096186));
#21818=CARTESIAN_POINT('Ctrl Pts',(5.6577376463315,2.74646568080389,7.83303706974588));
#21819=CARTESIAN_POINT('Ctrl Pts',(5.66743862330822,2.65313425633025,7.86508088454568));
#21820=CARTESIAN_POINT('Ctrl Pts',(5.66743862330822,2.47654785029388,7.92245728595387));
#21821=CARTESIAN_POINT('Ctrl Pts',(5.6577376463315,2.38220626001897,7.95139213009729));
#21822=CARTESIAN_POINT('Ctrl Pts',(5.63694838037124,2.28830166396294,7.97832535653344));
#21823=CARTESIAN_POINT('Ctrl Pts',(2.36305161962877,2.83826704815898,7.79963077096185));
#21824=CARTESIAN_POINT('Ctrl Pts',(2.56564497161068,2.77475170678765,7.61514961115078));
#21825=CARTESIAN_POINT('Ctrl Pts',(2.8414185613243,2.71625203654638,7.44544836653197));
#21826=CARTESIAN_POINT('Ctrl Pts',(3.36598484931781,2.64540317647514,7.24001881570869));
#21827=CARTESIAN_POINT('Ctrl Pts',(3.70875810561651,2.6231528858578,7.17556053123489));
#21828=CARTESIAN_POINT('Ctrl Pts',(4.29124189438349,2.6231528858578,7.17556053123489));
#21829=CARTESIAN_POINT('Ctrl Pts',(4.6340151506822,2.64540317647514,7.24001881570869));
#21830=CARTESIAN_POINT('Ctrl Pts',(5.1585814386757,2.71625203654638,7.44544836653197));
#21831=CARTESIAN_POINT('Ctrl Pts',(5.43435502838932,2.77475170678765,7.61514961115077));
#21832=CARTESIAN_POINT('Ctrl Pts',(5.63694838037123,2.83826704815898,7.79963077096185));
#21833=CARTESIAN_POINT('Origin',(4.,0.,0.));
#21834=CARTESIAN_POINT('',(2.36305161962877,9.25963747468151,7.15186086536041));
#21835=CARTESIAN_POINT('Origin',(2.36305161962877,0.,0.));
#21836=CARTESIAN_POINT('Ctrl Pts',(2.36305161962877,9.2596374746815,7.15186086536043));
#21837=CARTESIAN_POINT('Ctrl Pts',(2.56564335337965,9.41577612470673,7.26884057730416));
#21838=CARTESIAN_POINT('Ctrl Pts',(2.84141117550506,9.55944543027122,7.37642824958397));
#21839=CARTESIAN_POINT('Ctrl Pts',(3.36597543488952,9.73338541206091,7.5066654368745));
#21840=CARTESIAN_POINT('Ctrl Pts',(3.7087541062761,9.7879741784414,7.54752684540867));
#21841=CARTESIAN_POINT('Ctrl Pts',(4.,9.7879741784414,7.54752684540867));
#21842=CARTESIAN_POINT('Ctrl Pts',(4.2912458937239,9.7879741784414,7.54752684540867));
#21843=CARTESIAN_POINT('Ctrl Pts',(4.63402456511048,9.73338541206091,7.5066654368745));
#21844=CARTESIAN_POINT('Ctrl Pts',(5.15858882449494,9.55944543027121,7.37642824958397));
#21845=CARTESIAN_POINT('Ctrl Pts',(5.43435664662035,9.41577612470672,7.26884057730416));
#21846=CARTESIAN_POINT('Ctrl Pts',(5.63694838037123,9.2596374746815,7.15186086536043));
#21847=CARTESIAN_POINT('Origin',(4.,0.,0.));
#21848=CARTESIAN_POINT('',(5.63694838037123,6.54081691696393,5.10957082921437));
#21849=CARTESIAN_POINT('Origin',(5.63694838037123,0.,0.));
#21850=CARTESIAN_POINT('Ctrl Pts',(5.63694838037123,6.54081691696392,5.10957082921439));
#21851=CARTESIAN_POINT('Ctrl Pts',(5.43435502838932,6.38499222767917,4.99215633639486));
#21852=CARTESIAN_POINT('Ctrl Pts',(5.1585814386757,6.24167414543094,4.88407927525699));
#21853=CARTESIAN_POINT('Ctrl Pts',(4.63401515068219,6.06819253427498,4.75321678286295));
#21854=CARTESIAN_POINT('Ctrl Pts',(4.29124189438349,6.01376478072751,4.7121367936512));
#21855=CARTESIAN_POINT('Ctrl Pts',(3.70875810561651,6.01376478072751,4.7121367936512));
#21856=CARTESIAN_POINT('Ctrl Pts',(3.36598484931781,6.06819253427498,4.75321678286295));
#21857=CARTESIAN_POINT('Ctrl Pts',(2.8414185613243,6.24167414543094,4.88407927525699));
#21858=CARTESIAN_POINT('Ctrl Pts',(2.56564497161068,6.38499222767917,4.99215633639486));
#21859=CARTESIAN_POINT('Ctrl Pts',(2.36305161962877,6.54081691696392,5.10957082921439));
#21860=CARTESIAN_POINT('Origin',(4.,8.09016994374947,5.87785252292473));
#21861=CARTESIAN_POINT('',(4.,6.69050631172802,7.80432424078007));
#21862=CARTESIAN_POINT('',(4.,9.48983357577093,3.95138080506939));
#21863=CARTESIAN_POINT('Origin',(4.,8.09016994374947,5.87785252292473));
#21864=CARTESIAN_POINT('',(2.36305161962877,9.66320922106503,6.59639201002516));
#21865=CARTESIAN_POINT('Ctrl Pts',(2.36305161962877,9.66320922106503,6.59639201002516));
#21866=CARTESIAN_POINT('Ctrl Pts',(2.34215062955513,9.59746823296338,6.69269752392734));
#21867=CARTESIAN_POINT('Ctrl Pts',(2.33256137669178,9.53010584356091,6.78816353218381));
#21868=CARTESIAN_POINT('Ctrl Pts',(2.33256137669178,9.40089182481286,6.96601137146006));
#21869=CARTESIAN_POINT('Ctrl Pts',(2.34215062955512,9.33091437868292,7.05957742979088));
#21870=CARTESIAN_POINT('Ctrl Pts',(2.36305161962876,9.25963747468151,7.15186086536041));
#21871=CARTESIAN_POINT('Ctrl Pts',(5.63694838037123,9.66320922106504,6.59639201002515));
#21872=CARTESIAN_POINT('Ctrl Pts',(5.43435664662035,9.82271303472001,6.70873997158947));
#21873=CARTESIAN_POINT('Ctrl Pts',(5.15858882449494,9.96943124850423,6.81213118171848));
#21874=CARTESIAN_POINT('Ctrl Pts',(4.63402456511048,10.1470445845151,6.93731243067146));
#21875=CARTESIAN_POINT('Ctrl Pts',(4.2912458937239,10.2027749498801,6.97660256300298));
#21876=CARTESIAN_POINT('Ctrl Pts',(4.,10.2027749498801,6.97660256300298));
#21877=CARTESIAN_POINT('Ctrl Pts',(3.7087541062761,10.2027749498801,6.97660256300298));
#21878=CARTESIAN_POINT('Ctrl Pts',(3.36597543488952,10.1470445845151,6.93731243067146));
#21879=CARTESIAN_POINT('Ctrl Pts',(2.84141117550506,9.96943124850423,6.81213118171847));
#21880=CARTESIAN_POINT('Ctrl Pts',(2.56564335337965,9.82271303472001,6.70873997158947));
#21881=CARTESIAN_POINT('Ctrl Pts',(2.36305161962877,9.66320922106504,6.59639201002515));
#21882=CARTESIAN_POINT('',(5.63694838037123,6.88071421703297,4.64174233058239));
#21883=CARTESIAN_POINT('Ctrl Pts',(5.63694838037124,6.88071421703297,4.64174233058239));
#21884=CARTESIAN_POINT('Ctrl Pts',(5.6577376463315,6.82608108049478,4.72272808388943));
#21885=CARTESIAN_POINT('Ctrl Pts',(5.66743862330822,6.7694092537529,4.80351090950812));
#21886=CARTESIAN_POINT('Ctrl Pts',(5.66743862330822,6.66027285287123,4.95372427854694));
#21887=CARTESIAN_POINT('Ctrl Pts',(5.6577376463315,6.60095637772736,5.03258565462996));
#21888=CARTESIAN_POINT('Ctrl Pts',(5.63694838037124,6.54081691696393,5.10957082921437));
#21889=CARTESIAN_POINT('Ctrl Pts',(2.36305161962877,6.88071421703298,4.64174233058237));
#21890=CARTESIAN_POINT('Ctrl Pts',(2.56564497161068,6.72089392139729,4.5298273181056));
#21891=CARTESIAN_POINT('Ctrl Pts',(2.8414185613243,6.57381880512416,4.4269213706742));
#21892=CARTESIAN_POINT('Ctrl Pts',(3.36598484931781,6.39575241293544,4.30236928800296));
#21893=CARTESIAN_POINT('Ctrl Pts',(3.70875810561651,6.33986392069446,4.26329983311949));
#21894=CARTESIAN_POINT('Ctrl Pts',(4.29124189438349,6.33986392069446,4.26329983311949));
#21895=CARTESIAN_POINT('Ctrl Pts',(4.63401515068219,6.39575241293544,4.30236928800296));
#21896=CARTESIAN_POINT('Ctrl Pts',(5.1585814386757,6.57381880512416,4.4269213706742));
#21897=CARTESIAN_POINT('Ctrl Pts',(5.43435502838932,6.72089392139729,4.5298273181056));
#21898=CARTESIAN_POINT('Ctrl Pts',(5.63694838037123,6.88071421703298,4.64174233058237));
#21899=CARTESIAN_POINT('Origin',(1.18152580981438,0.,0.));
#21900=CARTESIAN_POINT('',(2.36305161962877,11.694962421875,-0.343298632289183));
#21901=CARTESIAN_POINT('Origin',(2.36305161962877,0.,0.));
#21902=CARTESIAN_POINT('',(2.36305161962877,11.694962421875,0.343298632289183));
#21903=CARTESIAN_POINT('Ctrl Pts',(2.36305161962876,11.694962421875,-0.343298632289183));
#21904=CARTESIAN_POINT('Ctrl Pts',(2.34215062955512,11.6983838060599,-0.226744251613026));
#21905=CARTESIAN_POINT('Ctrl Pts',(2.33256137669178,11.7,-0.109916009498452));
#21906=CARTESIAN_POINT('Ctrl Pts',(2.33256137669178,11.7,0.109916009498452));
#21907=CARTESIAN_POINT('Ctrl Pts',(2.34215062955512,11.6983838060599,0.226744251613026));
#21908=CARTESIAN_POINT('Ctrl Pts',(2.36305161962876,11.694962421875,0.343298632289183));
#21909=CARTESIAN_POINT('Origin',(2.36305161962877,0.,0.));
#21910=CARTESIAN_POINT('',(0.,-11.7,-1.4328367550024E-15));
#21911=CARTESIAN_POINT('',(1.18152580981438,-11.7,-1.4328367550024E-15));
#21912=CARTESIAN_POINT('Origin',(0.,0.,0.));
#21913=CARTESIAN_POINT('Origin',(4.,0.,0.));
#21914=CARTESIAN_POINT('Ctrl Pts',(5.63694838037123,11.694962421875,-0.3432986322892));
#21915=CARTESIAN_POINT('Ctrl Pts',(5.43435664662035,11.8900401927221,-0.346161211451081));
#21916=CARTESIAN_POINT('Ctrl Pts',(5.15858882449494,12.0695095495884,-0.348754767692784));
#21917=CARTESIAN_POINT('Ctrl Pts',(4.63402456511048,12.2867814488469,-0.351879509430406));
#21918=CARTESIAN_POINT('Ctrl Pts',(4.2912458937239,12.354962421875,-0.35285061152936));
#21919=CARTESIAN_POINT('Ctrl Pts',(4.,12.354962421875,-0.35285061152936));
#21920=CARTESIAN_POINT('Ctrl Pts',(3.7087541062761,12.354962421875,-0.35285061152936));
#21921=CARTESIAN_POINT('Ctrl Pts',(3.36597543488952,12.2867814488469,-0.351879509430406));
#21922=CARTESIAN_POINT('Ctrl Pts',(2.84141117550506,12.0695095495884,-0.348754767692784));
#21923=CARTESIAN_POINT('Ctrl Pts',(2.56564335337965,11.8900401927221,-0.346161211451081));
#21924=CARTESIAN_POINT('Ctrl Pts',(2.36305161962877,11.694962421875,-0.343298632289201));
#21925=CARTESIAN_POINT('Origin',(6.81847419018562,0.,0.));
#21926=CARTESIAN_POINT('',(8.,-8.3,-1.0164568432923E-15));
#21927=CARTESIAN_POINT('Origin',(8.,0.,0.));
#21928=CARTESIAN_POINT('',(6.81847419018562,-8.3,-1.0164568432923E-15));
#21929=CARTESIAN_POINT('',(5.63694838037123,8.294962421875,-0.289133913060399));
#21930=CARTESIAN_POINT('Origin',(5.63694838037123,0.,0.));
#21931=CARTESIAN_POINT('',(5.63694838037123,8.294962421875,0.289133913060399));
#21932=CARTESIAN_POINT('Ctrl Pts',(5.63694838037124,8.294962421875,-0.2891339130604));
#21933=CARTESIAN_POINT('Ctrl Pts',(5.6577376463315,8.29836551739928,-0.191502510389123));
#21934=CARTESIAN_POINT('Ctrl Pts',(5.66743862330822,8.3,-0.0928369676306243));
#21935=CARTESIAN_POINT('Ctrl Pts',(5.66743862330822,8.3,0.0928369676306244));
#21936=CARTESIAN_POINT('Ctrl Pts',(5.6577376463315,8.29836551739928,0.191502510389123));
#21937=CARTESIAN_POINT('Ctrl Pts',(5.63694838037124,8.294962421875,0.2891339130604));
#21938=CARTESIAN_POINT('Origin',(5.63694838037123,0.,0.));
#21939=CARTESIAN_POINT('Origin',(4.,0.,0.));
#21940=CARTESIAN_POINT('Ctrl Pts',(2.36305161962877,8.294962421875,-0.289133913060425));
#21941=CARTESIAN_POINT('Ctrl Pts',(2.56564497161068,8.09988309281573,-0.285735047288138));
#21942=CARTESIAN_POINT('Ctrl Pts',(2.8414185613243,7.92041022602773,-0.282539123257847));
#21943=CARTESIAN_POINT('Ctrl Pts',(3.36598484931781,7.70314161128355,-0.278639075566218));
#21944=CARTESIAN_POINT('Ctrl Pts',(3.70875810561651,7.634962421875,-0.277396497015792));
#21945=CARTESIAN_POINT('Ctrl Pts',(4.29124189438349,7.634962421875,-0.277396497015792));
#21946=CARTESIAN_POINT('Ctrl Pts',(4.63401515068219,7.70314161128355,-0.278639075566218));
#21947=CARTESIAN_POINT('Ctrl Pts',(5.1585814386757,7.92041022602772,-0.282539123257847));
#21948=CARTESIAN_POINT('Ctrl Pts',(5.43435502838932,8.09988309281573,-0.285735047288133));
#21949=CARTESIAN_POINT('Ctrl Pts',(5.63694838037123,8.294962421875,-0.289133913060422));
#21950=CARTESIAN_POINT('Origin',(4.,10.,0.));
#21951=CARTESIAN_POINT('',(4.,10.,2.38125));
#21952=CARTESIAN_POINT('',(4.,10.,-2.38125));
#21953=CARTESIAN_POINT('Origin',(4.,10.,0.));
#21954=CARTESIAN_POINT('Ctrl Pts',(5.63694838037123,8.294962421875,0.289133913060422));
#21955=CARTESIAN_POINT('Ctrl Pts',(5.43435502838932,8.09988309281573,0.285735047288134));
#21956=CARTESIAN_POINT('Ctrl Pts',(5.1585814386757,7.92041022602772,0.282539123257847));
#21957=CARTESIAN_POINT('Ctrl Pts',(4.63401515068219,7.70314161128355,0.278639075566218));
#21958=CARTESIAN_POINT('Ctrl Pts',(4.29124189438349,7.634962421875,0.277396497015792));
#21959=CARTESIAN_POINT('Ctrl Pts',(3.70875810561651,7.634962421875,0.277396497015792));
#21960=CARTESIAN_POINT('Ctrl Pts',(3.36598484931781,7.70314161128355,0.278639075566218));
#21961=CARTESIAN_POINT('Ctrl Pts',(2.8414185613243,7.92041022602773,0.282539123257847));
#21962=CARTESIAN_POINT('Ctrl Pts',(2.56564497161068,8.09988309281573,0.285735047288138));
#21963=CARTESIAN_POINT('Ctrl Pts',(2.36305161962877,8.294962421875,0.289133913060426));
#21964=CARTESIAN_POINT('Ctrl Pts',(2.36305161962877,11.694962421875,0.3432986322892));
#21965=CARTESIAN_POINT('Ctrl Pts',(2.56564335337965,11.8900401927221,0.346161211451081));
#21966=CARTESIAN_POINT('Ctrl Pts',(2.84141117550506,12.0695095495884,0.348754767692783));
#21967=CARTESIAN_POINT('Ctrl Pts',(3.36597543488952,12.2867814488469,0.351879509430406));
#21968=CARTESIAN_POINT('Ctrl Pts',(3.7087541062761,12.354962421875,0.35285061152936));
#21969=CARTESIAN_POINT('Ctrl Pts',(4.,12.354962421875,0.35285061152936));
#21970=CARTESIAN_POINT('Ctrl Pts',(4.2912458937239,12.354962421875,0.35285061152936));
#21971=CARTESIAN_POINT('Ctrl Pts',(4.63402456511048,12.2867814488469,0.351879509430406));
#21972=CARTESIAN_POINT('Ctrl Pts',(5.15858882449494,12.0695095495884,0.348754767692784));
#21973=CARTESIAN_POINT('Ctrl Pts',(5.43435664662035,11.8900401927221,0.34616121145108));
#21974=CARTESIAN_POINT('Ctrl Pts',(5.63694838037123,11.694962421875,0.343298632289199));
#21975=CARTESIAN_POINT('Origin',(4.,0.,0.));
#21976=CARTESIAN_POINT('Origin',(0.,13.7,0.));
#21977=CARTESIAN_POINT('',(3.81639164714898E-16,-13.7,-1.67776611483187E-15));
#21978=CARTESIAN_POINT('Origin',(0.,0.,0.));
#21979=CARTESIAN_POINT('Origin',(0.15,0.,0.));
#21980=CARTESIAN_POINT('',(0.300000000000001,-14.,-1.71450551880629E-15));
#21981=CARTESIAN_POINT('Origin',(0.3,0.,0.));
#21982=CARTESIAN_POINT('',(0.15,-13.85,-1.69613581681908E-15));
#21983=CARTESIAN_POINT('Origin',(4.,0.,0.));
#21984=CARTESIAN_POINT('',(7.7,-14.,-1.71450551880629E-15));
#21985=CARTESIAN_POINT('Origin',(7.7,0.,0.));
#21986=CARTESIAN_POINT('',(4.,-14.,-1.71450551880629E-15));
#21987=CARTESIAN_POINT('Origin',(7.85,0.,0.));
#21988=CARTESIAN_POINT('',(8.,-13.7,-1.67776611483187E-15));
#21989=CARTESIAN_POINT('Origin',(8.,0.,0.));
#21990=CARTESIAN_POINT('',(7.85,-13.85,-1.69613581681908E-15));
#21991=CARTESIAN_POINT('Origin',(8.,12.6,0.));
#21992=CARTESIAN_POINT('',(8.,-12.6,-1.54305496692567E-15));
#21993=CARTESIAN_POINT('Origin',(8.,0.,0.));
#21994=CARTESIAN_POINT('Origin',(7.1,0.,0.));
#21995=CARTESIAN_POINT('',(7.1,-12.6,-1.54305496692567E-15));
#21996=CARTESIAN_POINT('Origin',(4.,0.,0.));
#21997=CARTESIAN_POINT('Origin',(8.,6.3,0.));
#21998=CARTESIAN_POINT('',(8.,-6.3,-7.71527483462833E-16));
#21999=CARTESIAN_POINT('Origin',(8.,0.,0.));
#22000=CARTESIAN_POINT('Origin',(7.85,0.,0.));
#22001=CARTESIAN_POINT('',(7.7,-6.,-7.34788079488412E-16));
#22002=CARTESIAN_POINT('',(7.85,-6.15,-7.53157781475622E-16));
#22003=CARTESIAN_POINT('Origin',(7.7,0.,0.));
#22004=CARTESIAN_POINT('Origin',(4.,0.,0.));
#22005=CARTESIAN_POINT('',(0.3,-6.,-7.34788079488412E-16));
#22006=CARTESIAN_POINT('',(4.,-6.,-7.34788079488412E-16));
#22007=CARTESIAN_POINT('Origin',(0.3,0.,0.));
#22008=CARTESIAN_POINT('Origin',(0.15,0.,0.));
#22009=CARTESIAN_POINT('',(-6.93889390390723E-17,-6.3,-7.71527483462833E-16));
#22010=CARTESIAN_POINT('',(0.15,-6.15,-7.53157781475622E-16));
#22011=CARTESIAN_POINT('Origin',(0.,0.,0.));
#22012=CARTESIAN_POINT('Origin',(0.,8.3,0.));
#23237=UNCERTAINTY_MEASURE_WITH_UNIT(LENGTH_MEASURE(0.01),#23255,
'DISTANCE_ACCURACY_VALUE',
'Maximum model space distance between geometric entities at asserted c
onnectivities');
#23242=UNCERTAINTY_MEASURE_WITH_UNIT(LENGTH_MEASURE(0.01),#23255,
'DISTANCE_ACCURACY_VALUE',
'Maximum model space distance between geometric entities at asserted c
onnectivities');
#23249=(
GEOMETRIC_REPRESENTATION_CONTEXT(3)
GLOBAL_UNCERTAINTY_ASSIGNED_CONTEXT((#23237))
GLOBAL_UNIT_ASSIGNED_CONTEXT((#23255,#23257,#23258))
REPRESENTATION_CONTEXT('','3D')
);
#23254=(
GEOMETRIC_REPRESENTATION_CONTEXT(3)
GLOBAL_UNCERTAINTY_ASSIGNED_CONTEXT((#23242))
GLOBAL_UNIT_ASSIGNED_CONTEXT((#23255,#23257,#23258))
REPRESENTATION_CONTEXT('','3D')
);
#23255=(
LENGTH_UNIT()
NAMED_UNIT(*)
SI_UNIT(.MILLI.,.METRE.)
);
#23257=(
NAMED_UNIT(*)
PLANE_ANGLE_UNIT()
SI_UNIT($,.RADIAN.)
);
#23258=(
NAMED_UNIT(*)
SI_UNIT($,.STERADIAN.)
SOLID_ANGLE_UNIT()
);
#23265=SHAPE_DEFINITION_REPRESENTATION(#23276,#23305);
#23276=PRODUCT_DEFINITION_SHAPE('',$,#23317);
#23305=SHAPE_REPRESENTATION('',(#7604),#23249);
#23310=PRODUCT_DEFINITION_CONTEXT('part definition',#23345,'design');
#23317=PRODUCT_DEFINITION('2026-10-11-09-11-53-414',
'06_Angular_Contact_Ball_Bearing_7001_12x28x8',#23328,#23310);
#23328=PRODUCT_DEFINITION_FORMATION('',$,#23353);
#23345=APPLICATION_CONTEXT(
'Core Data for Automotive Mechanical Design Process');
#23346=PRODUCT_CONTEXT('part definition',#23345,'mechanical');
#23353=PRODUCT('2026-10-11-09-11-53-414',
'06_Angular_Contact_Ball_Bearing_7001_12x28x8',$,(#23346));
#23456=COLOUR_RGB('Grey',0.48,0.52,0.57);
#23457=FILL_AREA_STYLE_COLOUR('',#23456);
#23458=FILL_AREA_STYLE('',(#23457));
#23459=SURFACE_STYLE_FILL_AREA(#23458);
#23460=SURFACE_SIDE_STYLE('',(#23459));
#23461=SURFACE_STYLE_USAGE(.BOTH.,#23460);
#23462=PRESENTATION_STYLE_ASSIGNMENT((#23461));
ENDSEC;
END-ISO-10303-21;
